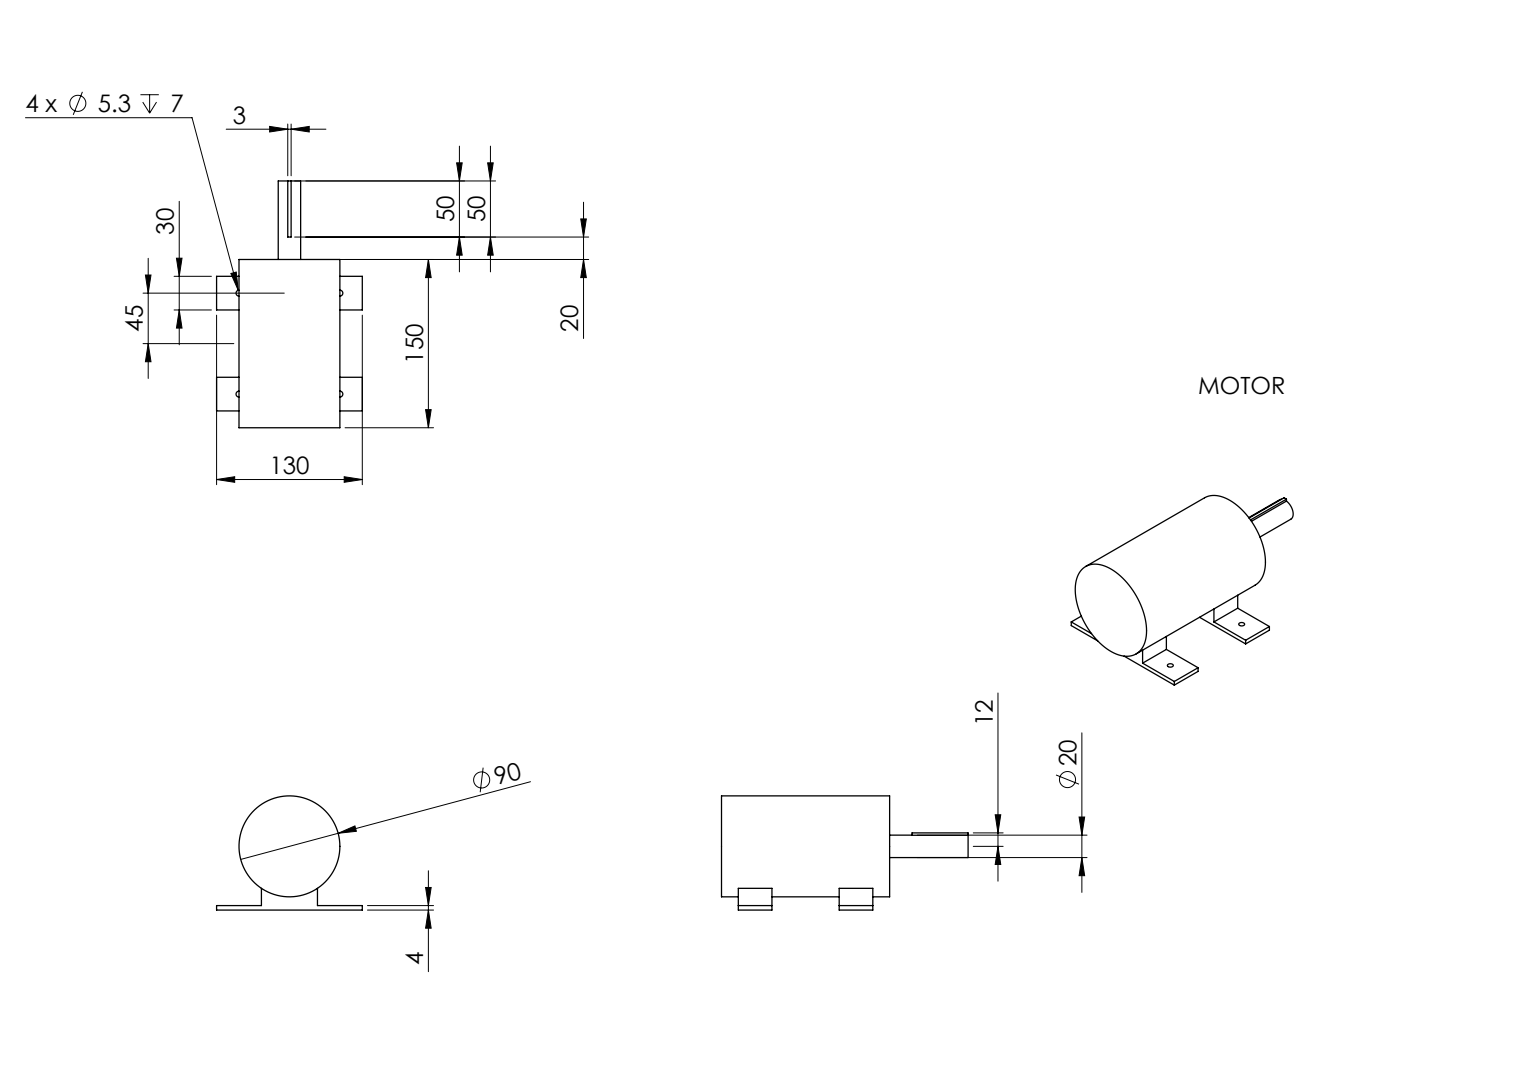
ISO-10303-21;
HEADER;
FILE_DESCRIPTION (('STEP AP214'),
    '1' );
FILE_NAME ('motor.step',
    '2026-10-31T03:46:07',
    ( '' ),
    ( '' ),
    'SwSTEP 2.0',
    'SolidWorks 2026',
    '' );
FILE_SCHEMA (( 'AUTOMOTIVE_DESIGN' ));
ENDSEC;

DATA;
#31=EDGE_CURVE ( 'NONE', #18619, #12627, #9184, .T. ) ;
#51=DIRECTION ( 'NONE',  ( -0.000000000000000000, 3.469446951953613794E-15, 1.000000000000000000 ) ) ;
#52=VERTEX_POINT ( 'NONE', #18122 ) ;
#60=EDGE_CURVE ( 'NONE', #21739, #840, #11018, .T. ) ;
#75=ORIENTED_EDGE ( 'NONE', *, *, #4902, .T. ) ;
#109=AXIS2_PLACEMENT_3D ( 'NONE', #8463, #1435, #15716 ) ;
#182=ADVANCED_FACE ( 'NONE', ( #22679 ), #11370, .F. ) ;
#186=DIRECTION ( 'NONE',  ( 0.000000000000000000, 0.000000000000000000, 1.000000000000000000 ) ) ;
#214=FACE_BOUND ( 'NONE', #6282, .T. ) ;
#228=CARTESIAN_POINT ( 'NONE',  ( -44.99999999999995026, -52.79999999999969873, 50.00000000000018474 ) ) ;
#267=EDGE_CURVE ( 'NONE', #8364, #19016, #14886, .T. ) ;
#271=EDGE_CURVE ( 'NONE', #15472, #22598, #15342, .T. ) ;
#296=VECTOR ( 'NONE', #1760, 1000.000000000000000 ) ;
#300=DIRECTION ( 'NONE',  ( 1.000000000000000000, 3.202566417187951028E-16, 6.405132834375902056E-16 ) ) ;
#324=DIRECTION ( 'NONE',  ( 0.000000000000000000, 0.000000000000000000, 1.000000000000000000 ) ) ;
#328=DIRECTION ( 'NONE',  ( 0.000000000000000000, 0.000000000000000000, 1.000000000000000000 ) ) ;
#332=ORIENTED_EDGE ( 'NONE', *, *, #16929, .T. ) ;
#347=LINE ( 'NONE', #14855, #18432 ) ;
#354=MECHANICAL_DESIGN_GEOMETRIC_PRESENTATION_REPRESENTATION('',(#10787),#11568);
#418=DIRECTION ( 'NONE',  ( 1.000000000000000000, 3.202566417187951028E-16, 6.405132834375902056E-16 ) ) ;
#436=VERTEX_POINT ( 'NONE', #17740 ) ;
#447=DIRECTION ( 'NONE',  ( 0.000000000000000000, 0.000000000000000000, 1.000000000000000000 ) ) ;
#475=CARTESIAN_POINT ( 'NONE',  ( -64.99999999999995737, -56.79999999999964899, 65.00000000000018474 ) ) ;
#486=VECTOR ( 'NONE', #22174, 1000.000000000000000 ) ;
#488=EDGE_CURVE ( 'NONE', #4511, #21370, #19433, .T. ) ;
#514=ORIENTED_EDGE ( 'NONE', *, *, #11865, .F. ) ;
#573=FACE_OUTER_BOUND ( 'NONE', #17478, .T. ) ;
#585=EDGE_CURVE ( 'NONE', #16285, #2501, #3259, .T. ) ;
#591=ORIENTED_EDGE ( 'NONE', *, *, #17311, .T. ) ;
#622=EDGE_LOOP ( 'NONE', ( #22663, #20160, #16621, #5819 ) ) ;
#695=AXIS2_PLACEMENT_3D ( 'NONE', #11043, #18024, #7144 ) ;
#700=ORIENTED_EDGE ( 'NONE', *, *, #8357, .T. ) ;
#712=LINE ( 'NONE', #4213, #4849 ) ;
#713=EDGE_CURVE ( 'NONE', #9956, #13794, #10236, .T. ) ;
#721=VECTOR ( 'NONE', #17814, 1000.000000000000000 ) ;
#731=ORIENTED_EDGE ( 'NONE', *, *, #5331, .T. ) ;
#753=UNCERTAINTY_MEASURE_WITH_UNIT (LENGTH_MEASURE( 1.000000000000000082E-05 ), #23433, 'distance_accuracy_value', 'NONE');
#754=FACE_OUTER_BOUND ( 'NONE', #19293, .T. ) ;
#786=LINE ( 'NONE', #9977, #23718 ) ;
#797=FACE_OUTER_BOUND ( 'NONE', #2972, .T. ) ;
#840=VERTEX_POINT ( 'NONE', #23717 ) ;
#894=DIRECTION ( 'NONE',  ( 0.000000000000000000, -1.000000000000000000, 3.392348130799088816E-15 ) ) ;
#943=ORIENTED_EDGE ( 'NONE', *, *, #1344, .F. ) ;
#989=DIRECTION ( 'NONE',  ( 0.000000000000000000, 0.000000000000000000, 1.000000000000000000 ) ) ;
#993=EDGE_LOOP ( 'NONE', ( #23590, #14200 ) ) ;
#1019=ORIENTED_EDGE ( 'NONE', *, *, #13645, .T. ) ;
#1061=EDGE_LOOP ( 'NONE', ( #11544, #14347, #943, #7992 ) ) ;
#1081=DIRECTION ( 'NONE',  ( 1.000000000000000000, 3.736327486719276364E-16, 1.067522139062650425E-16 ) ) ;
#1090=DIRECTION ( 'NONE',  ( 1.000000000000000000, 3.469446951953598905E-16, -4.625929269271499719E-16 ) ) ;
#1094=VECTOR ( 'NONE', #15458, 1000.000000000000000 ) ;
#1097=CARTESIAN_POINT ( 'NONE',  ( 25.00000000000001421, -37.41657386773940885, 125.0000000000001705 ) ) ;
#1101=DIRECTION ( 'NONE',  ( 3.202566417187928841E-16, -1.000000000000000000, 3.469446951953614583E-15 ) ) ;
#1155=ADVANCED_FACE ( 'NONE', ( #19690 ), #10664, .F. ) ;
#1156=VERTEX_POINT ( 'NONE', #21271 ) ;
#1180=CARTESIAN_POINT ( 'NONE',  ( 65.00000000000001421, -52.79999999999938609, 125.0000000000002274 ) ) ;
#1201=CARTESIAN_POINT ( 'NONE',  ( -44.99999999999995026, -52.79999999999969162, 52.65000000000017621 ) ) ;
#1218=ADVANCED_FACE ( 'NONE', ( #7472 ), #7018, .T. ) ;
#1228=DIRECTION ( 'NONE',  ( -0.000000000000000000, -0.000000000000000000, -1.000000000000000000 ) ) ;
#1234=ORIENTED_EDGE ( 'NONE', *, *, #20465, .F. ) ;
#1239=DIRECTION ( 'NONE',  ( 0.000000000000000000, 2.618450529776326854E-15, 1.000000000000000000 ) ) ;
#1245=DIRECTION ( 'NONE',  ( 3.736327486719275871E-16, -1.000000000000000000, 3.469446951953613794E-15 ) ) ;
#1257=VERTEX_POINT ( 'NONE', #22201 ) ;
#1270=CARTESIAN_POINT ( 'NONE',  ( 1.500000000000000000, 0.000000000000000000, 0.000000000000000000 ) ) ;
#1273=FACE_OUTER_BOUND ( 'NONE', #8704, .T. ) ;
#1277=VERTEX_POINT ( 'NONE', #3856 ) ;
#1292=ORIENTED_EDGE ( 'NONE', *, *, #17778, .T. ) ;
#1324=ORIENTED_EDGE ( 'NONE', *, *, #4746, .T. ) ;
#1344=EDGE_CURVE ( 'NONE', #18619, #4703, #7733, .T. ) ;
#1346=EDGE_CURVE ( 'NONE', #19016, #7096, #712, .T. ) ;
#1353=EDGE_LOOP ( 'NONE', ( #21943, #75 ) ) ;
#1376=ADVANCED_FACE ( 'NONE', ( #19177 ), #11869, .T. ) ;
#1379=ADVANCED_FACE ( 'NONE', ( #11635 ), #2640, .F. ) ;
#1417=PLANE ( 'NONE',  #12387 ) ;
#1424=ORIENTED_EDGE ( 'NONE', *, *, #19677, .F. ) ;
#1425=VECTOR ( 'NONE', #2146, 1000.000000000000000 ) ;
#1426=CARTESIAN_POINT ( 'NONE',  ( 25.00000000000004263, -37.41657386773938754, 65.00000000000018474 ) ) ;
#1435=DIRECTION ( 'NONE',  ( 0.000000000000000000, 0.000000000000000000, 1.000000000000000000 ) ) ;
#1443=EDGE_CURVE ( 'NONE', #4246, #14920, #21250, .T. ) ;
#1489=ORIENTED_EDGE ( 'NONE', *, *, #11624, .T. ) ;
#1499=AXIS2_PLACEMENT_3D ( 'NONE', #3288, #4753, #2922 ) ;
#1592=VERTEX_POINT ( 'NONE', #1660 ) ;
#1593=ORIENTED_EDGE ( 'NONE', *, *, #2778, .F. ) ;
#1610=CARTESIAN_POINT ( 'NONE',  ( -44.99999999999997868, -52.79999999999939320, 137.3500000000001648 ) ) ;
#1639=EDGE_CURVE ( 'NONE', #1592, #2833, #13352, .T. ) ;
#1660=CARTESIAN_POINT ( 'NONE',  ( 45.00000000000002132, -56.79999999999935767, 137.3500000000002217 ) ) ;
#1662=AXIS2_PLACEMENT_3D ( 'NONE', #5057, #9144, #22047 ) ;
#1664=EDGE_CURVE ( 'NONE', #21370, #4532, #16298, .T. ) ;
#1673=CARTESIAN_POINT ( 'NONE',  ( 45.00000000000004974, -52.79999999999967741, 47.35000000000018616 ) ) ;
#1691=LINE ( 'NONE', #1933, #20050 ) ;
#1707=CARTESIAN_POINT ( 'NONE',  ( -44.99999999999997868, -52.79999999999938609, 140.0000000000001421 ) ) ;
#1752=CIRCLE ( 'NONE', #22195, 2.649999999999999467 ) ;
#1759=CARTESIAN_POINT ( 'NONE',  ( -1.500000000000000000, 12.00000000000000000, -50.00000000000000000 ) ) ;
#1760=DIRECTION ( 'NONE',  ( -1.000000000000000000, 0.000000000000000000, 0.000000000000000000 ) ) ;
#1789=PRODUCT_DEFINITION_CONTEXT ( 'detailed design', #19235, 'design' ) ;
#1792=CARTESIAN_POINT ( 'NONE',  ( -44.99999999999995026, -52.79999999999969873, 50.00000000000018474 ) ) ;
#1800=ADVANCED_FACE ( 'NONE', ( #214, #573 ), #4314, .F. ) ;
#1808=CYLINDRICAL_SURFACE ( 'NONE', #23222, 2.649999999999999467 ) ;
#1813=DIRECTION ( 'NONE',  ( 1.751623080406021339E-46, 3.469446951953613794E-15, 1.000000000000000000 ) ) ;
#1828=LINE ( 'NONE', #5350, #21940 ) ;
#1839=CARTESIAN_POINT ( 'NONE',  ( -1.500000000000000000, 9.886859966642592923, -50.00000000000000000 ) ) ;
#1849=CARTESIAN_POINT ( 'NONE',  ( 45.00000000000000711, 5.510910596163090344E-15, 169.9999999999999716 ) ) ;
#1863=AXIS2_PLACEMENT_3D ( 'NONE', #5506, #11334, #20339 ) ;
#1865=LINE ( 'NONE', #21914, #7643 ) ;
#1875=ORIENTED_EDGE ( 'NONE', *, *, #2102, .F. ) ;
#1895=CARTESIAN_POINT ( 'NONE',  ( 45.00000000000004974, -52.79999999999966320, 52.65000000000017621 ) ) ;
#1905=ADVANCED_FACE ( 'NONE', ( #1273 ), #8190, .F. ) ;
#1933=CARTESIAN_POINT ( 'NONE',  ( -24.99999999999995381, -52.79999999999975557, 35.00000000000017764 ) ) ;
#1940=EDGE_CURVE ( 'NONE', #10258, #9956, #8997, .T. ) ;
#1943=LINE ( 'NONE', #5686, #11472 ) ;
#1968=CARTESIAN_POINT ( 'NONE',  ( 45.00000000000002132, -52.79999999999935767, 142.6500000000002046 ) ) ;
#2007=DIRECTION ( 'NONE',  ( 0.000000000000000000, -3.469446951953613794E-15, -1.000000000000000000 ) ) ;
#2016=VECTOR ( 'NONE', #23551, 1000.000000000000000 ) ;
#2045=DIRECTION ( 'NONE',  ( 0.000000000000000000, 2.618450529776313049E-15, 1.000000000000000000 ) ) ;
#2057=AXIS2_PLACEMENT_3D ( 'NONE', #14966, #22065, #4060 ) ;
#2074=ORIENTED_EDGE ( 'NONE', *, *, #31, .T. ) ;
#2102=EDGE_CURVE ( 'NONE', #10287, #52, #11208, .T. ) ;
#2145=CARTESIAN_POINT ( 'NONE',  ( 0.000000000000000000, 0.000000000000000000, 155.0000000000000284 ) ) ;
#2146=DIRECTION ( 'NONE',  ( 1.751623080406021339E-46, 3.469446951953613794E-15, 1.000000000000000000 ) ) ;
#2152=CYLINDRICAL_SURFACE ( 'NONE', #19096, 2.649999999999999467 ) ;
#2168=CARTESIAN_POINT ( 'NONE',  ( 45.00000000000004974, -52.79999999999966320, 52.65000000000018332 ) ) ;
#2206=AXIS2_PLACEMENT_3D ( 'NONE', #13977, #1245, #21179 ) ;
#2244=EDGE_LOOP ( 'NONE', ( #17085, #2250, #21077, #7054 ) ) ;
#2250=ORIENTED_EDGE ( 'NONE', *, *, #14976, .F. ) ;
#2322=PRODUCT_DEFINITION_FORMATION_WITH_SPECIFIED_SOURCE ( 'ANY', '', #3218, .NOT_KNOWN. ) ;
#2366=CARTESIAN_POINT ( 'NONE',  ( 25.00000000000002132, -52.79999999999942162, 125.0000000000001990 ) ) ;
#2398=DIRECTION ( 'NONE',  ( 3.736327486719275871E-16, -1.000000000000000000, 3.469446951953614189E-15 ) ) ;
#2436=DIRECTION ( 'NONE',  ( -0.000000000000000000, 1.000000000000000000, -3.469446951953613794E-15 ) ) ;
#2437=EDGE_LOOP ( 'NONE', ( #12043, #17343, #8968, #13517, #4232, #20219, #1875, #17937 ) ) ;
#2464=CIRCLE ( 'NONE', #9037, 2.649999999999985700 ) ;
#2465=DIRECTION ( 'NONE',  ( -1.000000000000000000, -3.202566417187951028E-16, -6.405132834375902056E-16 ) ) ;
#2501=VERTEX_POINT ( 'NONE', #20080 ) ;
#2505=FACE_OUTER_BOUND ( 'NONE', #10784, .T. ) ;
#2522=DIRECTION ( 'NONE',  ( 0.000000000000000000, 0.000000000000000000, 1.000000000000000000 ) ) ;
#2528=EDGE_LOOP ( 'NONE', ( #23738, #21267 ) ) ;
#2614=DIRECTION ( 'NONE',  ( -4.625929269271485914E-16, -3.469446951953614583E-15, -1.000000000000000000 ) ) ;
#2633=ORIENTED_EDGE ( 'NONE', *, *, #5098, .T. ) ;
#2637=CARTESIAN_POINT ( 'NONE',  ( -24.99999999999998579, -37.41657386773942306, 169.9999999999999716 ) ) ;
#2640=PLANE ( 'NONE',  #17162 ) ;
#2658=EDGE_CURVE ( 'NONE', #2501, #12643, #22364, .T. ) ;
#2679=ORIENTED_EDGE ( 'NONE', *, *, #6053, .T. ) ;
#2694=AXIS2_PLACEMENT_3D ( 'NONE', #9686, #4584, #15123 ) ;
#2762=DIRECTION ( 'NONE',  ( -0.000000000000000000, 1.000000000000000000, -3.469446951953613794E-15 ) ) ;
#2766=DIRECTION ( 'NONE',  ( -0.000000000000000000, 1.000000000000000000, -3.469446951953613794E-15 ) ) ;
#2778=EDGE_CURVE ( 'NONE', #4532, #8574, #10433, .T. ) ;
#2833=VERTEX_POINT ( 'NONE', #14730 ) ;
#2836=DIRECTION ( 'NONE',  ( 0.000000000000000000, -2.618450529776313049E-15, -1.000000000000000000 ) ) ;
#2885=ORIENTED_EDGE ( 'NONE', *, *, #22707, .F. ) ;
#2898=DIRECTION ( 'NONE',  ( 0.000000000000000000, -2.618450529776326854E-15, -1.000000000000000000 ) ) ;
#2899=CARTESIAN_POINT ( 'NONE',  ( 25.00000000000004974, -52.79999999999973426, 35.00000000000017764 ) ) ;
#2918=CARTESIAN_POINT ( 'NONE',  ( -1.500000000000000000, 12.00000000000000000, 0.000000000000000000 ) ) ;
#2920=EDGE_CURVE ( 'NONE', #1277, #23309, #20491, .T. ) ;
#2922=DIRECTION ( 'NONE',  ( -1.000000000000000000, 0.000000000000000000, 0.000000000000000000 ) ) ;
#2941=ORIENTED_EDGE ( 'NONE', *, *, #10411, .F. ) ;
#2972=EDGE_LOOP ( 'NONE', ( #19259, #16489, #3704, #1292 ) ) ;
#2979=DIRECTION ( 'NONE',  ( 2.238759164535664589E-46, 3.469446951953614189E-15, 1.000000000000000000 ) ) ;
#2982=VERTEX_POINT ( 'NONE', #18663 ) ;
#2991=CARTESIAN_POINT ( 'NONE',  ( 1.500000000000000000, 12.00000000000000000, 0.000000000000000000 ) ) ;
#3005=AXIS2_PLACEMENT_3D ( 'NONE', #7570, #5878, #2007 ) ;
#3007=CIRCLE ( 'NONE', #23458, 2.649999999999999467 ) ;
#3045=DIRECTION ( 'NONE',  ( 0.000000000000000000, 0.000000000000000000, 1.000000000000000000 ) ) ;
#3113=VERTEX_POINT ( 'NONE', #8546 ) ;
#3124=SHAPE_REPRESENTATION ( 'motor', ( #11210 ), #7665 ) ;
#3189=DIRECTION ( 'NONE',  ( 3.736327486719275871E-16, -1.000000000000000000, 3.469446951953613794E-15 ) ) ;
#3218=PRODUCT ( 'motor', 'motor', '', ( #7579 ) ) ;
#3234=ORIENTED_EDGE ( 'NONE', *, *, #21969, .F. ) ;
#3247=CARTESIAN_POINT ( 'NONE',  ( -24.99999999999998934, 45.00100000000031031, 34.99999999999983658 ) ) ;
#3254=DIRECTION ( 'NONE',  ( -0.000000000000000000, 1.000000000000000000, -3.469446951953613794E-15 ) ) ;
#3259=CIRCLE ( 'NONE', #12952, 45.00000000000000711 ) ;
#3272=CIRCLE ( 'NONE', #16782, 45.00000000000000711 ) ;
#3281=CYLINDRICAL_SURFACE ( 'NONE', #20382, 45.00000000000000711 ) ;
#3288=CARTESIAN_POINT ( 'NONE',  ( 0.000000000000000000, 0.000000000000000000, 169.9999999999999716 ) ) ;
#3294=DIRECTION ( 'NONE',  ( 1.000000000000000000, 0.000000000000000000, 0.000000000000000000 ) ) ;
#3296=LINE ( 'NONE', #1610, #20557 ) ;
#3309=EDGE_LOOP ( 'NONE', ( #10169, #7031, #1019, #15364 ) ) ;
#3310=ADVANCED_FACE ( 'NONE', ( #23331 ), #14321, .F. ) ;
#3324=ORIENTED_EDGE ( 'NONE', *, *, #3934, .T. ) ;
#3334=ADVANCED_FACE ( 'NONE', ( #23094 ), #12517, .T. ) ;
#3365=ADVANCED_FACE ( 'NONE', ( #4743 ), #3281, .T. ) ;
#3374=ADVANCED_FACE ( 'NONE', ( #12272 ), #10198, .F. ) ;
#3382=AXIS2_PLACEMENT_3D ( 'NONE', #13638, #9741, #894 ) ;
#3415=VERTEX_POINT ( 'NONE', #23246 ) ;
#3427=VECTOR ( 'NONE', #7829, 1000.000000000000000 ) ;
#3495=SURFACE_STYLE_USAGE ( .BOTH. , #5756 ) ;
#3528=ORIENTED_EDGE ( 'NONE', *, *, #4495, .F. ) ;
#3529=DIRECTION ( 'NONE',  ( 3.736327486719275871E-16, -1.000000000000000000, 3.469446951953613794E-15 ) ) ;
#3538=EDGE_CURVE ( 'NONE', #12643, #17916, #11599, .T. ) ;
#3565=EDGE_LOOP ( 'NONE', ( #5410, #19936, #9737, #16180 ) ) ;
#3574=EDGE_CURVE ( 'NONE', #8832, #13580, #22258, .T. ) ;
#3575=ORIENTED_EDGE ( 'NONE', *, *, #7698, .T. ) ;
#3578=EDGE_LOOP ( 'NONE', ( #16303, #3575, #14895, #19374 ) ) ;
#3589=DIRECTION ( 'NONE',  ( -0.000000000000000000, 1.000000000000000000, -3.469446951953613794E-15 ) ) ;
#3592=CARTESIAN_POINT ( 'NONE',  ( 65.00000000000004263, -52.79999999999959925, 65.00000000000018474 ) ) ;
#3594=VECTOR ( 'NONE', #20916, 1000.000000000000000 ) ;
#3673=AXIS2_PLACEMENT_3D ( 'NONE', #18231, #10908, #20269 ) ;
#3681=ORIENTED_EDGE ( 'NONE', *, *, #22989, .F. ) ;
#3695=CARTESIAN_POINT ( 'NONE',  ( 45.00000000000002132, -56.79999999999935056, 140.0000000000001990 ) ) ;
#3704=ORIENTED_EDGE ( 'NONE', *, *, #713, .T. ) ;
#3719=CARTESIAN_POINT ( 'NONE',  ( 65.00000000000005684, -52.79999999999970584, 35.00000000000017764 ) ) ;
#3724=EDGE_LOOP ( 'NONE', ( #11287, #11752 ) ) ;
#3744=ORIENTED_EDGE ( 'NONE', *, *, #7934, .F. ) ;
#3768=CARTESIAN_POINT ( 'NONE',  ( 45.00000000000002132, -52.79999999999936477, 137.3500000000002217 ) ) ;
#3769=DIRECTION ( 'NONE',  ( 1.000000000000000000, 0.000000000000000000, 0.000000000000000000 ) ) ;
#3773=CARTESIAN_POINT ( 'NONE',  ( -44.99999999999997868, -56.79999999999937188, 142.6500000000001478 ) ) ;
#3786=ORIENTED_EDGE ( 'NONE', *, *, #6661, .T. ) ;
#3789=DIRECTION ( 'NONE',  ( 0.000000000000000000, 0.000000000000000000, 1.000000000000000000 ) ) ;
#3840=VECTOR ( 'NONE', #7258, 1000.000000000000000 ) ;
#3847=ADVANCED_FACE ( 'NONE', ( #12418, #10696, #21659 ), #5115, .T. ) ;
#3853=CARTESIAN_POINT ( 'NONE',  ( 25.00000000000002132, -52.79999999999942162, 125.0000000000001990 ) ) ;
#3856=CARTESIAN_POINT ( 'NONE',  ( 65.00000000000002842, -52.79999999999929372, 155.0000000000002274 ) ) ;
#3881=EDGE_LOOP ( 'NONE', ( #19327, #2633, #15079, #19810 ) ) ;
#3924=SHAPE_REPRESENTATION_RELATIONSHIP ( 'NONE' , 'NONE' ,  #3124, #22256 ) ;
#3928=EDGE_CURVE ( 'NONE', #12485, #6553, #1828, .T. ) ;
#3934=EDGE_CURVE ( 'NONE', #12627, #22432, #11178, .T. ) ;
#3962=FACE_OUTER_BOUND ( 'NONE', #3881, .T. ) ;
#3963=EDGE_CURVE ( 'NONE', #8364, #436, #7509, .T. ) ;
#3986=VECTOR ( 'NONE', #10399, 1000.000000000000000 ) ;
#4058=AXIS2_PLACEMENT_3D ( 'NONE', #14297, #1090, #15857 ) ;
#4060=DIRECTION ( 'NONE',  ( 0.000000000000000000, 2.618450529776326854E-15, 1.000000000000000000 ) ) ;
#4078=DIRECTION ( 'NONE',  ( -2.238759164535664589E-46, -3.469446951953614189E-15, -1.000000000000000000 ) ) ;
#4142=VERTEX_POINT ( 'NONE', #23428 ) ;
#4193=ORIENTED_EDGE ( 'NONE', *, *, #9622, .T. ) ;
#4213=CARTESIAN_POINT ( 'NONE',  ( -25.00000000000001776, 45.00100000000072953, 154.9999999999998579 ) ) ;
#4226=AXIS2_PLACEMENT_3D ( 'NONE', #20020, #12709, #7213 ) ;
#4227=CARTESIAN_POINT ( 'NONE',  ( -64.99999999999998579, -52.79999999999942872, 125.0000000000001421 ) ) ;
#4232=ORIENTED_EDGE ( 'NONE', *, *, #11663, .T. ) ;
#4244=CIRCLE ( 'NONE', #5411, 2.649999999999985700 ) ;
#4246=VERTEX_POINT ( 'NONE', #1097 ) ;
#4254=ADVANCED_FACE ( 'NONE', ( #23197 ), #12254, .T. ) ;
#4307=LINE ( 'NONE', #16859, #6183 ) ;
#4312=DIRECTION ( 'NONE',  ( 1.000000000000000000, 0.000000000000000000, 0.000000000000000000 ) ) ;
#4314=PLANE ( 'NONE',  #3005 ) ;
#4382=ORIENTED_EDGE ( 'NONE', *, *, #488, .T. ) ;
#4398=EDGE_LOOP ( 'NONE', ( #9314, #14380, #9069, #16829 ) ) ;
#4423=CARTESIAN_POINT ( 'NONE',  ( 25.00000000000001066, 45.00100000000033162, 34.99999999999983658 ) ) ;
#4442=AXIS2_PLACEMENT_3D ( 'NONE', #18688, #9678, #7963 ) ;
#4458=CARTESIAN_POINT ( 'NONE',  ( -65.00000000000000000, -56.79999999999932925, 155.0000000000001705 ) ) ;
#4459=ORIENTED_EDGE ( 'NONE', *, *, #3574, .T. ) ;
#4467=ADVANCED_FACE ( 'NONE', ( #3962 ), #2152, .F. ) ;
#4479=AXIS2_PLACEMENT_3D ( 'NONE', #20915, #2436, #9708 ) ;
#4495=EDGE_CURVE ( 'NONE', #1277, #5510, #21124, .T. ) ;
#4511=VERTEX_POINT ( 'NONE', #15480 ) ;
#4531=CARTESIAN_POINT ( 'NONE',  ( 1.500000000000000000, 12.00000000000000000, 0.000000000000000000 ) ) ;
#4532=VERTEX_POINT ( 'NONE', #1201 ) ;
#4541=DIRECTION ( 'NONE',  ( 1.000000000000000000, 0.000000000000000000, 0.000000000000000000 ) ) ;
#4552=EDGE_CURVE ( 'NONE', #12588, #21739, #12230, .T. ) ;
#4584=DIRECTION ( 'NONE',  ( 3.736327486719275871E-16, -1.000000000000000000, 3.469446951953613794E-15 ) ) ;
#4605=LINE ( 'NONE', #6411, #8756 ) ;
#4619=CARTESIAN_POINT ( 'NONE',  ( -24.99999999999996092, -37.41657386773943728, 35.00000000000013500 ) ) ;
#4640=DIRECTION ( 'NONE',  ( -0.000000000000000000, -0.000000000000000000, -1.000000000000000000 ) ) ;
#4650=AXIS2_PLACEMENT_3D ( 'NONE', #228, #13301, #6137 ) ;
#4683=LINE ( 'NONE', #13900, #23065 ) ;
#4703=VERTEX_POINT ( 'NONE', #1426 ) ;
#4713=CARTESIAN_POINT ( 'NONE',  ( -64.99999999999995737, -52.79999999999965610, 65.00000000000017053 ) ) ;
#4714=( LENGTH_UNIT ( ) NAMED_UNIT ( * ) SI_UNIT ( .MILLI., .METRE. ) );
#4743=FACE_OUTER_BOUND ( 'NONE', #20923, .T. ) ;
#4744=DIRECTION ( 'NONE',  ( -1.000000000000000000, 0.000000000000000000, 0.000000000000000000 ) ) ;
#4746=EDGE_CURVE ( 'NONE', #2501, #16285, #3272, .T. ) ;
#4753=DIRECTION ( 'NONE',  ( -0.000000000000000000, -0.000000000000000000, -1.000000000000000000 ) ) ;
#4761=EDGE_CURVE ( 'NONE', #15959, #10287, #786, .T. ) ;
#4788=CARTESIAN_POINT ( 'NONE',  ( 45.00000000000004974, -56.79999999999966320, 52.65000000000019753 ) ) ;
#4797=DIRECTION ( 'NONE',  ( -1.000000000000000000, -3.469446951953630952E-16, -4.625929269271472109E-16 ) ) ;
#4804=ORIENTED_EDGE ( 'NONE', *, *, #19808, .T. ) ;
#4818=DIRECTION ( 'NONE',  ( 0.000000000000000000, 2.618450529776313049E-15, 1.000000000000000000 ) ) ;
#4832=FACE_OUTER_BOUND ( 'NONE', #20243, .T. ) ;
#4849=VECTOR ( 'NONE', #8099, 1000.000000000000000 ) ;
#4850=CARTESIAN_POINT ( 'NONE',  ( -64.99999999999997158, -52.79999999999974847, 35.00000000000017764 ) ) ;
#4869=CARTESIAN_POINT ( 'NONE',  ( 1.500000000000000000, 0.000000000000000000, 0.000000000000000000 ) ) ;
#4873=LINE ( 'NONE', #2918, #21876 ) ;
#4874=ORIENTED_EDGE ( 'NONE', *, *, #10945, .T. ) ;
#4880=CARTESIAN_POINT ( 'NONE',  ( -24.99999999999998579, -37.41657386773942306, 155.0000000000001705 ) ) ;
#4902=EDGE_CURVE ( 'NONE', #13580, #4142, #13759, .T. ) ;
#4903=VECTOR ( 'NONE', #2398, 1000.000000000000000 ) ;
#4956=AXIS2_PLACEMENT_3D ( 'NONE', #15563, #22889, #6357 ) ;
#4972=AXIS2_PLACEMENT_3D ( 'NONE', #19995, #6732, #9025 ) ;
#5013=ORIENTED_EDGE ( 'NONE', *, *, #13507, .F. ) ;
#5017=VECTOR ( 'NONE', #17639, 1000.000000000000000 ) ;
#5057=CARTESIAN_POINT ( 'NONE',  ( 0.000000000000000000, 0.000000000000000000, 0.000000000000000000 ) ) ;
#5058=VERTEX_POINT ( 'NONE', #21773 ) ;
#5098=EDGE_CURVE ( 'NONE', #23584, #18606, #1752, .T. ) ;
#5109=DIRECTION ( 'NONE',  ( 1.000000000000000000, 0.000000000000000000, 0.000000000000000000 ) ) ;
#5115=CYLINDRICAL_SURFACE ( 'NONE', #1499, 45.00000000000000711 ) ;
#5118=CIRCLE ( 'NONE', #12495, 2.649999999999985700 ) ;
#5180=DIRECTION ( 'NONE',  ( 3.469446951953614682E-16, -1.000000000000000000, 3.483493295888648978E-15 ) ) ;
#5192=EDGE_CURVE ( 'NONE', #13453, #2982, #16348, .T. ) ;
#5195=ORIENTED_EDGE ( 'NONE', *, *, #31, .F. ) ;
#5196=ADVANCED_FACE ( 'NONE', ( #754 ), #13714, .F. ) ;
#5205=VECTOR ( 'NONE', #8406, 1000.000000000000000 ) ;
#5232=ADVANCED_FACE ( 'NONE', ( #18970 ), #7881, .F. ) ;
#5241=ORIENTED_EDGE ( 'NONE', *, *, #2778, .T. ) ;
#5322=EDGE_CURVE ( 'NONE', #9373, #8692, #4244, .T. ) ;
#5331=EDGE_CURVE ( 'NONE', #21739, #12627, #10554, .T. ) ;
#5350=CARTESIAN_POINT ( 'NONE',  ( -24.99999999999998934, 45.00100000000031031, 34.99999999999983658 ) ) ;
#5410=ORIENTED_EDGE ( 'NONE', *, *, #23493, .T. ) ;
#5411=AXIS2_PLACEMENT_3D ( 'NONE', #8487, #1101, #2898 ) ;
#5414=CARTESIAN_POINT ( 'NONE',  ( 1.500000000000000000, 12.00000000000000000, -50.00000000000000000 ) ) ;
#5434=CARTESIAN_POINT ( 'NONE',  ( 45.00000000000002132, -56.79999999999935056, 140.0000000000001990 ) ) ;
#5463=ORIENTED_EDGE ( 'NONE', *, *, #14844, .T. ) ;
#5506=CARTESIAN_POINT ( 'NONE',  ( 0.000000000000000000, 0.000000000000000000, -50.00000000000000000 ) ) ;
#5510=VERTEX_POINT ( 'NONE', #13088 ) ;
#5514=EDGE_CURVE ( 'NONE', #13453, #19560, #18478, .T. ) ;
#5579=EDGE_CURVE ( 'NONE', #6553, #21767, #1691, .T. ) ;
#5681=FACE_OUTER_BOUND ( 'NONE', #14860, .T. ) ;
#5684=CARTESIAN_POINT ( 'NONE',  ( -24.99999999999995381, -52.79999999999965610, 65.00000000000018474 ) ) ;
#5686=CARTESIAN_POINT ( 'NONE',  ( -24.99999999999998224, -52.79999999999944293, 125.0000000000001990 ) ) ;
#5695=EDGE_LOOP ( 'NONE', ( #20282, #23163 ) ) ;
#5708=CARTESIAN_POINT ( 'NONE',  ( -64.99999999999997158, -56.79999999999975557, 35.00000000000019185 ) ) ;
#5753=AXIS2_PLACEMENT_3D ( 'NONE', #17540, #989, #12411 ) ;
#5756=SURFACE_SIDE_STYLE ('',( #15605 ) ) ;
#5764=CIRCLE ( 'NONE', #19246, 45.00000000000000711 ) ;
#5793=VECTOR ( 'NONE', #23523, 1000.000000000000000 ) ;
#5819=ORIENTED_EDGE ( 'NONE', *, *, #7398, .T. ) ;
#5870=DIRECTION ( 'NONE',  ( 1.000000000000000000, 3.736327486719276364E-16, 1.067522139062650425E-16 ) ) ;
#5878=DIRECTION ( 'NONE',  ( 3.736327486719275871E-16, -1.000000000000000000, 3.469446951953613794E-15 ) ) ;
#5881=ORIENTED_EDGE ( 'NONE', *, *, #17201, .F. ) ;
#5884=CARTESIAN_POINT ( 'NONE',  ( 65.00000000000001421, -52.79999999999938609, 125.0000000000002274 ) ) ;
#5902=DIRECTION ( 'NONE',  ( -0.000000000000000000, 1.000000000000000000, -3.469446951953613794E-15 ) ) ;
#5911=PLANE ( 'NONE',  #2694 ) ;
#5937=AXIS2_PLACEMENT_3D ( 'NONE', #16851, #5982, #9380 ) ;
#5975=DIRECTION ( 'NONE',  ( 1.000000000000000000, 0.000000000000000000, 0.000000000000000000 ) ) ;
#5982=DIRECTION ( 'NONE',  ( 3.202566417187928841E-16, -1.000000000000000000, 3.469446951953614583E-15 ) ) ;
#5995=PLANE ( 'NONE',  #15078 ) ;
#6010=AXIS2_PLACEMENT_3D ( 'NONE', #15147, #20796, #13353 ) ;
#6026=DIRECTION ( 'NONE',  ( 1.000000000000000000, 3.469446951953630952E-16, 4.625929269271474081E-16 ) ) ;
#6028=EDGE_LOOP ( 'NONE', ( #514, #6048 ) ) ;
#6048=ORIENTED_EDGE ( 'NONE', *, *, #23000, .F. ) ;
#6053=EDGE_CURVE ( 'NONE', #8574, #4532, #13948, .T. ) ;
#6094=ADVANCED_FACE ( 'NONE', ( #18795 ), #6372, .F. ) ;
#6099=ORIENTED_EDGE ( 'NONE', *, *, #2102, .T. ) ;
#6137=DIRECTION ( 'NONE',  ( 0.000000000000000000, 2.618450529776319755E-15, 1.000000000000000000 ) ) ;
#6139=DIRECTION ( 'NONE',  ( 0.000000000000000000, 2.618450529776313049E-15, 1.000000000000000000 ) ) ;
#6150=DIRECTION ( 'NONE',  ( 0.000000000000000000, 2.618450529776326854E-15, 1.000000000000000000 ) ) ;
#6183=VECTOR ( 'NONE', #5870, 1000.000000000000000 ) ;
#6199=CARTESIAN_POINT ( 'NONE',  ( -44.99999999999997868, -52.79999999999938609, 140.0000000000001421 ) ) ;
#6271=ORIENTED_EDGE ( 'NONE', *, *, #19425, .T. ) ;
#6276=CARTESIAN_POINT ( 'NONE',  ( 25.00000000000004263, -37.41657386773938754, 169.9999999999999716 ) ) ;
#6282=EDGE_LOOP ( 'NONE', ( #17146, #18799 ) ) ;
#6298=ORIENTED_EDGE ( 'NONE', *, *, #7394, .T. ) ;
#6307=DIRECTION ( 'NONE',  ( 0.000000000000000000, 2.618450529776326854E-15, 1.000000000000000000 ) ) ;
#6357=DIRECTION ( 'NONE',  ( 0.000000000000000000, 0.000000000000000000, -1.000000000000000000 ) ) ;
#6371=AXIS2_PLACEMENT_3D ( 'NONE', #3695, #20015, #11109 ) ;
#6372=PLANE ( 'NONE',  #20441 ) ;
#6396=CARTESIAN_POINT ( 'NONE',  ( -64.99999999999995737, -52.79999999999965610, 65.00000000000017053 ) ) ;
#6411=CARTESIAN_POINT ( 'NONE',  ( -64.99999999999997158, -52.79999999999974847, 35.00000000000017764 ) ) ;
#6483=DIRECTION ( 'NONE',  ( -0.000000000000000000, 1.000000000000000000, -3.469446951953613794E-15 ) ) ;
#6486=FACE_OUTER_BOUND ( 'NONE', #622, .T. ) ;
#6499=ORIENTED_EDGE ( 'NONE', *, *, #1639, .T. ) ;
#6524=ORIENTED_EDGE ( 'NONE', *, *, #13507, .T. ) ;
#6526=DIRECTION ( 'NONE',  ( 0.000000000000000000, 1.000000000000000000, -3.469446951953614189E-15 ) ) ;
#6548=ORIENTED_EDGE ( 'NONE', *, *, #21176, .F. ) ;
#6550=( NAMED_UNIT ( * ) PLANE_ANGLE_UNIT ( ) SI_UNIT ( $, .RADIAN. ) );
#6552=DIRECTION ( 'NONE',  ( -0.000000000000000000, 1.000000000000000000, -3.469446951953613794E-15 ) ) ;
#6553=VERTEX_POINT ( 'NONE', #22273 ) ;
#6564=CARTESIAN_POINT ( 'NONE',  ( 45.00000000000002132, -52.79999999999936477, 137.3500000000002217 ) ) ;
#6612=ADVANCED_FACE ( 'NONE', ( #19130, #6669 ), #12262, .F. ) ;
#6647=DIRECTION ( 'NONE',  ( 0.000000000000000000, 0.000000000000000000, 1.000000000000000000 ) ) ;
#6650=DIRECTION ( 'NONE',  ( -2.238759164535664589E-46, -3.469446951953614189E-15, -1.000000000000000000 ) ) ;
#6661=EDGE_CURVE ( 'NONE', #16285, #17916, #11817, .T. ) ;
#6669=FACE_OUTER_BOUND ( 'NONE', #3565, .T. ) ;
#6673=DIRECTION ( 'NONE',  ( 0.000000000000000000, 0.000000000000000000, 1.000000000000000000 ) ) ;
#6685=DIRECTION ( 'NONE',  ( 0.000000000000000000, 0.000000000000000000, -1.000000000000000000 ) ) ;
#6691=DIRECTION ( 'NONE',  ( 1.000000000000000000, 3.202566417187951028E-16, 6.405132834375902056E-16 ) ) ;
#6732=DIRECTION ( 'NONE',  ( 1.000000000000000000, 3.736327486719275871E-16, -1.296299001029869881E-30 ) ) ;
#6738=CARTESIAN_POINT ( 'NONE',  ( -10.00000000000000000, 1.224646799147353256E-15, -50.00000000000000000 ) ) ;
#6762=ADVANCED_FACE ( 'NONE', ( #5681 ), #1808, .F. ) ;
#6855=FACE_OUTER_BOUND ( 'NONE', #20374, .T. ) ;
#6880=( NAMED_UNIT ( * ) PLANE_ANGLE_UNIT ( ) SI_UNIT ( $, .RADIAN. ) );
#6896=ADVANCED_FACE ( 'NONE', ( #20598, #13053, #10887 ), #9291, .T. ) ;
#6959=AXIS2_PLACEMENT_3D ( 'NONE', #7930, #328, #4541 ) ;
#6964=ORIENTED_EDGE ( 'NONE', *, *, #8123, .F. ) ;
#6973=CARTESIAN_POINT ( 'NONE',  ( 65.00000000000001421, -56.79999999999939320, 125.0000000000002558 ) ) ;
#6978=EDGE_CURVE ( 'NONE', #1156, #17333, #16869, .T. ) ;
#7011=( NAMED_UNIT ( * ) PLANE_ANGLE_UNIT ( ) SI_UNIT ( $, .RADIAN. ) );
#7017=ORIENTED_EDGE ( 'NONE', *, *, #6053, .F. ) ;
#7018=PLANE ( 'NONE',  #3673 ) ;
#7026=DIRECTION ( 'NONE',  ( 3.736327486719275871E-16, -1.000000000000000000, 3.469446951953613794E-15 ) ) ;
#7027=VERTEX_POINT ( 'NONE', #15564 ) ;
#7031=ORIENTED_EDGE ( 'NONE', *, *, #12434, .T. ) ;
#7043=ORIENTED_EDGE ( 'NONE', *, *, #11624, .F. ) ;
#7054=ORIENTED_EDGE ( 'NONE', *, *, #12443, .F. ) ;
#7080=CARTESIAN_POINT ( 'NONE',  ( -44.99999999999997868, -52.79999999999938609, 140.0000000000001421 ) ) ;
#7096=VERTEX_POINT ( 'NONE', #17239 ) ;
#7101=DIRECTION ( 'NONE',  ( -0.000000000000000000, 1.000000000000000000, -3.469446951953613794E-15 ) ) ;
#7131=EDGE_LOOP ( 'NONE', ( #8931, #4459, #7234, #21617, #12795, #17739, #16675, #15139 ) ) ;
#7144=DIRECTION ( 'NONE',  ( 1.000000000000000000, 0.000000000000000000, 0.000000000000000000 ) ) ;
#7172=ADVANCED_FACE ( 'NONE', ( #10414 ), #17870, .T. ) ;
#7213=DIRECTION ( 'NONE',  ( 0.000000000000000000, 2.618450529776319755E-15, 1.000000000000000000 ) ) ;
#7227=ADVANCED_FACE ( 'NONE', ( #10653, #17991 ), #14159, .F. ) ;
#7230=EDGE_CURVE ( 'NONE', #10258, #8832, #20149, .T. ) ;
#7234=ORIENTED_EDGE ( 'NONE', *, *, #10226, .F. ) ;
#7258=DIRECTION ( 'NONE',  ( -4.625929269271485914E-16, 3.469446951953614583E-15, 1.000000000000000000 ) ) ;
#7286=VECTOR ( 'NONE', #19741, 1000.000000000000000 ) ;
#7309=AXIS2_PLACEMENT_3D ( 'NONE', #4869, #4744, #3045 ) ;
#7310=ORIENTED_EDGE ( 'NONE', *, *, #5331, .F. ) ;
#7362=CARTESIAN_POINT ( 'NONE',  ( -44.99999999999995026, -52.79999999999970584, 47.35000000000019327 ) ) ;
#7379=DIRECTION ( 'NONE',  ( 3.736327486719275871E-16, -1.000000000000000000, 3.469446951953614189E-15 ) ) ;
#7394=EDGE_CURVE ( 'NONE', #2833, #1592, #5118, .T. ) ;
#7397=ORIENTED_EDGE ( 'NONE', *, *, #271, .T. ) ;
#7398=EDGE_CURVE ( 'NONE', #12588, #3415, #14612, .T. ) ;
#7400=DIRECTION ( 'NONE',  ( 3.736327486719275871E-16, -1.000000000000000000, 3.469446951953614189E-15 ) ) ;
#7406=EDGE_CURVE ( 'NONE', #23584, #7027, #14739, .T. ) ;
#7430=ADVANCED_FACE ( 'NONE', ( #2505 ), #13564, .F. ) ;
#7459=SHAPE_DEFINITION_REPRESENTATION ( #9034, #3124 ) ;
#7472=FACE_OUTER_BOUND ( 'NONE', #17508, .T. ) ;
#7496=ORIENTED_EDGE ( 'NONE', *, *, #12731, .T. ) ;
#7509=LINE ( 'NONE', #20431, #22316 ) ;
#7510=ORIENTED_EDGE ( 'NONE', *, *, #17353, .F. ) ;
#7537=DIRECTION ( 'NONE',  ( 1.000000000000000000, 0.000000000000000000, 0.000000000000000000 ) ) ;
#7570=CARTESIAN_POINT ( 'NONE',  ( 1.983456134378398743E-14, -52.79999999999986215, 1.831306136874101694E-13 ) ) ;
#7571=CARTESIAN_POINT ( 'NONE',  ( 1.819057724962738742E-14, -56.79999999999984794, 1.970645868709647811E-13 ) ) ;
#7579=PRODUCT_CONTEXT ( 'NONE', #16775, 'mechanical' ) ;
#7643=VECTOR ( 'NONE', #12564, 1000.000000000000000 ) ;
#7648=CIRCLE ( 'NONE', #14618, 45.00000000000000711 ) ;
#7658=EDGE_LOOP ( 'NONE', ( #21127, #22080, #14017, #17202 ) ) ;
#7665=( GEOMETRIC_REPRESENTATION_CONTEXT ( 3 ) GLOBAL_UNCERTAINTY_ASSIGNED_CONTEXT ( ( #22193 ) ) GLOBAL_UNIT_ASSIGNED_CONTEXT ( ( #4714, #6880, #19797 ) ) REPRESENTATION_CONTEXT ( 'NONE', 'WORKASPACE' ) );
#7677=DIRECTION ( 'NONE',  ( -1.000000000000000000, 0.000000000000000000, 0.000000000000000000 ) ) ;
#7695=AXIS2_PLACEMENT_3D ( 'NONE', #18397, #186, #7537 ) ;
#7698=EDGE_CURVE ( 'NONE', #9956, #11870, #15957, .T. ) ;
#7733=LINE ( 'NONE', #6276, #15284 ) ;
#7740=ORIENTED_EDGE ( 'NONE', *, *, #7398, .F. ) ;
#7764=DIRECTION ( 'NONE',  ( -0.000000000000000000, -0.000000000000000000, -1.000000000000000000 ) ) ;
#7829=DIRECTION ( 'NONE',  ( 4.625929269271486900E-16, 3.469446951953614978E-15, 1.000000000000000000 ) ) ;
#7853=STYLED_ITEM('',(#23934),#12608);
#7870=VECTOR ( 'NONE', #12210, 1000.000000000000000 ) ;
#7881=CYLINDRICAL_SURFACE ( 'NONE', #4479, 2.649999999999985700 ) ;
#7924=LINE ( 'NONE', #9634, #11600 ) ;
#7927=VECTOR ( 'NONE', #13927, 1000.000000000000000 ) ;
#7930=CARTESIAN_POINT ( 'NONE',  ( 0.000000000000000000, 0.000000000000000000, 20.00000000000000000 ) ) ;
#7934=EDGE_CURVE ( 'NONE', #3113, #13794, #23358, .T. ) ;
#7947=ORIENTED_EDGE ( 'NONE', *, *, #12443, .T. ) ;
#7953=CARTESIAN_POINT ( 'NONE',  ( 45.00000000000004974, -52.79999999999967031, 50.00000000000018474 ) ) ;
#7963=DIRECTION ( 'NONE',  ( 1.000000000000000000, 0.000000000000000000, -0.000000000000000000 ) ) ;
#7981=ORIENTED_EDGE ( 'NONE', *, *, #12731, .F. ) ;
#7992=ORIENTED_EDGE ( 'NONE', *, *, #13629, .F. ) ;
#8088=AXIS2_PLACEMENT_3D ( 'NONE', #16090, #10676, #8726 ) ;
#8099=DIRECTION ( 'NONE',  ( 3.736327486719275871E-16, -1.000000000000000000, 3.469446951953614189E-15 ) ) ;
#8100=ORIENTED_EDGE ( 'NONE', *, *, #16929, .F. ) ;
#8103=CARTESIAN_POINT ( 'NONE',  ( 45.00000000000004974, -52.79999999999967031, 50.00000000000018474 ) ) ;
#8109=FACE_OUTER_BOUND ( 'NONE', #17856, .T. ) ;
#8123=EDGE_CURVE ( 'NONE', #18606, #21871, #22096, .T. ) ;
#8189=EDGE_CURVE ( 'NONE', #15959, #7096, #1943, .T. ) ;
#8190=PLANE ( 'NONE',  #4956 ) ;
#8226=FILL_AREA_STYLE ('',( #10417 ) ) ;
#8269=EDGE_LOOP ( 'NONE', ( #10486, #22728, #10878, #14473 ) ) ;
#8277=AXIS2_PLACEMENT_3D ( 'NONE', #20506, #5902, #6150 ) ;
#8357=EDGE_CURVE ( 'NONE', #19560, #21767, #21371, .T. ) ;
#8364=VERTEX_POINT ( 'NONE', #23296 ) ;
#8366=ADVANCED_FACE ( 'NONE', ( #4832 ), #14290, .T. ) ;
#8381=DIRECTION ( 'NONE',  ( 2.238759164535664589E-46, 3.469446951953614189E-15, 1.000000000000000000 ) ) ;
#8406=DIRECTION ( 'NONE',  ( 0.000000000000000000, 1.000000000000000000, 0.000000000000000000 ) ) ;
#8426=CARTESIAN_POINT ( 'NONE',  ( 65.00000000000004263, -52.79999999999959925, 65.00000000000018474 ) ) ;
#8438=AXIS2_PLACEMENT_3D ( 'NONE', #13273, #7677, #447 ) ;
#8452=DIRECTION ( 'NONE',  ( 4.625929269271484928E-16, -3.469446951953613794E-15, -1.000000000000000000 ) ) ;
#8463=CARTESIAN_POINT ( 'NONE',  ( 0.000000000000000000, 0.000000000000000000, -50.00000000000000000 ) ) ;
#8487=CARTESIAN_POINT ( 'NONE',  ( -44.99999999999997868, -56.79999999999937899, 140.0000000000001421 ) ) ;
#8488=( NAMED_UNIT ( * ) SI_UNIT ( $, .STERADIAN. ) SOLID_ANGLE_UNIT ( ) );
#8527=CARTESIAN_POINT ( 'NONE',  ( 25.00000000000001421, -37.41657386773940885, 169.9999999999999716 ) ) ;
#8546=CARTESIAN_POINT ( 'NONE',  ( 1.500000000000000000, 12.00000000000000000, 0.000000000000000000 ) ) ;
#8563=ORIENTED_EDGE ( 'NONE', *, *, #8189, .T. ) ;
#8574=VERTEX_POINT ( 'NONE', #7362 ) ;
#8590=DIRECTION ( 'NONE',  ( -1.000000000000000000, -3.736327486719275871E-16, -0.000000000000000000 ) ) ;
#8596=ORIENTED_EDGE ( 'NONE', *, *, #16136, .T. ) ;
#8603=CARTESIAN_POINT ( 'NONE',  ( 45.00000000000004974, -56.79999999999967031, 50.00000000000019895 ) ) ;
#8616=PLANE ( 'NONE',  #7309 ) ;
#8638=DIRECTION ( 'NONE',  ( -1.000000000000000000, 0.000000000000000000, 0.000000000000000000 ) ) ;
#8647=CARTESIAN_POINT ( 'NONE',  ( -44.99999999999995026, -56.79999999999969873, 50.00000000000019895 ) ) ;
#8692=VERTEX_POINT ( 'NONE', #22672 ) ;
#8704=EDGE_LOOP ( 'NONE', ( #19337, #13827, #3744, #1489 ) ) ;
#8726=DIRECTION ( 'NONE',  ( 0.000000000000000000, -3.469446951953614583E-15, -1.000000000000000000 ) ) ;
#8756=VECTOR ( 'NONE', #8590, 1000.000000000000000 ) ;
#8832=VERTEX_POINT ( 'NONE', #6738 ) ;
#8868=DIRECTION ( 'NONE',  ( -1.000000000000000000, 0.000000000000000000, 0.000000000000000000 ) ) ;
#8895=ORIENTED_EDGE ( 'NONE', *, *, #2658, .F. ) ;
#8931=ORIENTED_EDGE ( 'NONE', *, *, #7230, .T. ) ;
#8944=CARTESIAN_POINT ( 'NONE',  ( 0.000000000000000000, 0.000000000000000000, 169.9999999999999716 ) ) ;
#8955=( NAMED_UNIT ( * ) SI_UNIT ( $, .STERADIAN. ) SOLID_ANGLE_UNIT ( ) );
#8968=ORIENTED_EDGE ( 'NONE', *, *, #1443, .T. ) ;
#8997=LINE ( 'NONE', #1839, #20031 ) ;
#9025=DIRECTION ( 'NONE',  ( -3.736327486719275871E-16, 1.000000000000000000, 0.000000000000000000 ) ) ;
#9034=PRODUCT_DEFINITION_SHAPE ( 'NONE', 'NONE',  #12164 ) ;
#9037=AXIS2_PLACEMENT_3D ( 'NONE', #7080, #19993, #10618 ) ;
#9069=ORIENTED_EDGE ( 'NONE', *, *, #12569, .T. ) ;
#9081=LINE ( 'NONE', #16440, #18099 ) ;
#9130=DIRECTION ( 'NONE',  ( 0.000000000000000000, 0.000000000000000000, 1.000000000000000000 ) ) ;
#9134=ORIENTED_EDGE ( 'NONE', *, *, #5322, .F. ) ;
#9144=DIRECTION ( 'NONE',  ( -0.000000000000000000, -0.000000000000000000, -1.000000000000000000 ) ) ;
#9173=LINE ( 'NONE', #475, #3427 ) ;
#9184=LINE ( 'NONE', #12846, #23327 ) ;
#9227=DIRECTION ( 'NONE',  ( 3.736327486719275871E-16, -1.000000000000000000, 3.469446951953614189E-15 ) ) ;
#9291=PLANE ( 'NONE',  #23605 ) ;
#9314=ORIENTED_EDGE ( 'NONE', *, *, #12434, .F. ) ;
#9353=CARTESIAN_POINT ( 'NONE',  ( -64.99999999999997158, -52.79999999999974847, 35.00000000000017764 ) ) ;
#9358=DIRECTION ( 'NONE',  ( 0.000000000000000000, 0.000000000000000000, 1.000000000000000000 ) ) ;
#9373=VERTEX_POINT ( 'NONE', #3773 ) ;
#9380=DIRECTION ( 'NONE',  ( 0.000000000000000000, -3.469446951953614583E-15, -1.000000000000000000 ) ) ;
#9473=CARTESIAN_POINT ( 'NONE',  ( 0.000000000000000000, 0.000000000000000000, 0.000000000000000000 ) ) ;
#9490=DIRECTION ( 'NONE',  ( 1.000000000000000000, 0.000000000000000000, 0.000000000000000000 ) ) ;
#9565=ORIENTED_EDGE ( 'NONE', *, *, #585, .T. ) ;
#9569=DIRECTION ( 'NONE',  ( 0.000000000000000000, 2.618450529776326854E-15, 1.000000000000000000 ) ) ;
#9622=EDGE_CURVE ( 'NONE', #1592, #21376, #23088, .T. ) ;
#9634=CARTESIAN_POINT ( 'NONE',  ( 10.00000000000000000, 0.000000000000000000, -50.00000000000000000 ) ) ;
#9637=ORIENTED_EDGE ( 'NONE', *, *, #6978, .T. ) ;
#9642=VECTOR ( 'NONE', #1228, 1000.000000000000000 ) ;
#9644=VECTOR ( 'NONE', #300, 1000.000000000000000 ) ;
#9658=LINE ( 'NONE', #22664, #1094 ) ;
#9678=DIRECTION ( 'NONE',  ( 0.000000000000000000, 0.000000000000000000, 1.000000000000000000 ) ) ;
#9686=CARTESIAN_POINT ( 'NONE',  ( 1.983456134378398743E-14, -52.79999999999986215, 1.831306136874101694E-13 ) ) ;
#9708=DIRECTION ( 'NONE',  ( 0.000000000000000000, 2.618450529776326854E-15, 1.000000000000000000 ) ) ;
#9719=EDGE_CURVE ( 'NONE', #52, #17333, #20071, .T. ) ;
#9737=ORIENTED_EDGE ( 'NONE', *, *, #11263, .T. ) ;
#9741=DIRECTION ( 'NONE',  ( -2.238759164535664589E-46, -3.469446951953614189E-15, -1.000000000000000000 ) ) ;
#9782=ORIENTED_EDGE ( 'NONE', *, *, #22707, .T. ) ;
#9908=CARTESIAN_POINT ( 'NONE',  ( 1.500000000000000000, 0.000000000000000000, -50.00000000000000000 ) ) ;
#9926=ADVANCED_FACE ( 'NONE', ( #6855 ), #1417, .T. ) ;
#9956=VERTEX_POINT ( 'NONE', #12580 ) ;
#9977=CARTESIAN_POINT ( 'NONE',  ( -64.99999999999998579, -52.79999999999942872, 125.0000000000001421 ) ) ;
#10040=DIRECTION ( 'NONE',  ( 0.000000000000000000, 0.000000000000000000, 1.000000000000000000 ) ) ;
#10042=DIRECTION ( 'NONE',  ( 4.625929269271474081E-16, 0.000000000000000000, -1.000000000000000000 ) ) ;
#10114=CARTESIAN_POINT ( 'NONE',  ( 45.00000000000004974, -56.79999999999967741, 47.35000000000020037 ) ) ;
#10155=CARTESIAN_POINT ( 'NONE',  ( 65.00000000000004263, -52.79999999999959925, 65.00000000000018474 ) ) ;
#10166=VERTEX_POINT ( 'NONE', #1759 ) ;
#10169=ORIENTED_EDGE ( 'NONE', *, *, #5322, .T. ) ;
#10177=CARTESIAN_POINT ( 'NONE',  ( -25.00000000000001776, 45.00100000000062295, 124.9999999999998579 ) ) ;
#10198=PLANE ( 'NONE',  #5753 ) ;
#10226=EDGE_CURVE ( 'NONE', #4142, #13580, #23474, .T. ) ;
#10235=ADVANCED_FACE ( 'NONE', ( #21083 ), #5995, .T. ) ;
#10236=LINE ( 'NONE', #22783, #5205 ) ;
#10237=AXIS2_PLACEMENT_3D ( 'NONE', #10177, #17521, #12391 ) ;
#10258=VERTEX_POINT ( 'NONE', #17361 ) ;
#10272=VECTOR ( 'NONE', #23697, 1000.000000000000000 ) ;
#10287=VERTEX_POINT ( 'NONE', #15558 ) ;
#10302=VECTOR ( 'NONE', #1081, 1000.000000000000000 ) ;
#10321=FACE_BOUND ( 'NONE', #18423, .T. ) ;
#10399=DIRECTION ( 'NONE',  ( 0.000000000000000000, 0.000000000000000000, -1.000000000000000000 ) ) ;
#10411=EDGE_CURVE ( 'NONE', #11870, #3113, #12440, .T. ) ;
#10414=FACE_OUTER_BOUND ( 'NONE', #3578, .T. ) ;
#10417=FILL_AREA_STYLE_COLOUR ( '', #21165 ) ;
#10433=CIRCLE ( 'NONE', #4226, 2.649999999999992806 ) ;
#10440=CARTESIAN_POINT ( 'NONE',  ( 45.00000000000000711, 5.510910596163090344E-15, 169.9999999999999716 ) ) ;
#10455=CARTESIAN_POINT ( 'NONE',  ( 0.000000000000000000, 0.000000000000000000, -50.00000000000000000 ) ) ;
#10486=ORIENTED_EDGE ( 'NONE', *, *, #19677, .T. ) ;
#10554=LINE ( 'NONE', #4850, #5017 ) ;
#10618=DIRECTION ( 'NONE',  ( 0.000000000000000000, 2.618450529776326854E-15, 1.000000000000000000 ) ) ;
#10653=FACE_BOUND ( 'NONE', #1353, .T. ) ;
#10664=PLANE ( 'NONE',  #4058 ) ;
#10669=EDGE_LOOP ( 'NONE', ( #19915, #22319, #6548, #13891 ) ) ;
#10676=DIRECTION ( 'NONE',  ( 3.202566417187928841E-16, -1.000000000000000000, 3.469446951953614583E-15 ) ) ;
#10677=ADVANCED_FACE ( 'NONE', ( #21174 ), #8616, .F. ) ;
#10690=DIRECTION ( 'NONE',  ( -0.000000000000000000, 1.000000000000000000, -3.469446951953613794E-15 ) ) ;
#10696=FACE_BOUND ( 'NONE', #1061, .T. ) ;
#10739=AXIS2_PLACEMENT_3D ( 'NONE', #18104, #12589, #21827 ) ;
#10748=LINE ( 'NONE', #5414, #296 ) ;
#10774=PRESENTATION_STYLE_ASSIGNMENT (( #3495 ) ) ;
#10781=FACE_OUTER_BOUND ( 'NONE', #23305, .T. ) ;
#10784=EDGE_LOOP ( 'NONE', ( #14748, #17992, #591, #6964 ) ) ;
#10787=STYLED_ITEM ( 'NONE', ( #10774 ), #22256 ) ;
#10795=AXIS2_PLACEMENT_3D ( 'NONE', #17796, #10690, #1239 ) ;
#10830=VECTOR ( 'NONE', #20893, 1000.000000000000000 ) ;
#10838=CARTESIAN_POINT ( 'NONE',  ( 1.500000000000000000, 12.00000000000000000, -50.00000000000000000 ) ) ;
#10875=ORIENTED_EDGE ( 'NONE', *, *, #17351, .T. ) ;
#10878=ORIENTED_EDGE ( 'NONE', *, *, #2920, .F. ) ;
#10887=FACE_OUTER_BOUND ( 'NONE', #15008, .T. ) ;
#10888=ORIENTED_EDGE ( 'NONE', *, *, #14712, .F. ) ;
#10904=DIRECTION ( 'NONE',  ( 3.469446951953614682E-16, -1.000000000000000000, 3.483493295888648978E-15 ) ) ;
#10907=ORIENTED_EDGE ( 'NONE', *, *, #19759, .T. ) ;
#10908=DIRECTION ( 'NONE',  ( 2.238759164535664589E-46, 3.469446951953614189E-15, 1.000000000000000000 ) ) ;
#10933=EDGE_CURVE ( 'NONE', #13544, #15472, #16194, .T. ) ;
#10938=ORIENTED_EDGE ( 'NONE', *, *, #23482, .F. ) ;
#10945=EDGE_CURVE ( 'NONE', #1156, #7096, #14813, .T. ) ;
#11010=CARTESIAN_POINT ( 'NONE',  ( 45.00000000000002132, -52.79999999999936477, 140.0000000000001990 ) ) ;
#11018=LINE ( 'NONE', #3719, #22911 ) ;
#11042=CARTESIAN_POINT ( 'NONE',  ( -64.99999999999998579, -56.79999999999943583, 125.0000000000001705 ) ) ;
#11043=CARTESIAN_POINT ( 'NONE',  ( 0.000000000000000000, 0.000000000000000000, -50.00000000000000000 ) ) ;
#11109=DIRECTION ( 'NONE',  ( 0.000000000000000000, -2.618450529776326854E-15, -1.000000000000000000 ) ) ;
#11152=CIRCLE ( 'NONE', #11944, 2.649999999999985700 ) ;
#11178=LINE ( 'NONE', #16702, #16937 ) ;
#11208=LINE ( 'NONE', #14925, #19916 ) ;
#11210=AXIS2_PLACEMENT_3D ( 'NONE', #9473, #14914, #3769 ) ;
#11226=EDGE_CURVE ( 'NONE', #5058, #4246, #14854, .T. ) ;
#11263=EDGE_CURVE ( 'NONE', #436, #1277, #21416, .T. ) ;
#11284=DIRECTION ( 'NONE',  ( -0.000000000000000000, 1.000000000000000000, -3.469446951953613794E-15 ) ) ;
#11287=ORIENTED_EDGE ( 'NONE', *, *, #13790, .F. ) ;
#11334=DIRECTION ( 'NONE',  ( 0.000000000000000000, 0.000000000000000000, 1.000000000000000000 ) ) ;
#11337=ORIENTED_EDGE ( 'NONE', *, *, #19808, .F. ) ;
#11361=ORIENTED_EDGE ( 'NONE', *, *, #5192, .F. ) ;
#11370=CYLINDRICAL_SURFACE ( 'NONE', #8277, 2.649999999999985700 ) ;
#11408=CARTESIAN_POINT ( 'NONE',  ( -45.00000000000000711, 0.000000000000000000, 169.9999999999999716 ) ) ;
#11451=DIRECTION ( 'NONE',  ( -1.000000000000000000, -3.202566417187951028E-16, -6.405132834375902056E-16 ) ) ;
#11472=VECTOR ( 'NONE', #1813, 1000.000000000000000 ) ;
#11544=ORIENTED_EDGE ( 'NONE', *, *, #13943, .T. ) ;
#11568=( GEOMETRIC_REPRESENTATION_CONTEXT ( 3 ) GLOBAL_UNCERTAINTY_ASSIGNED_CONTEXT ( ( #14745 ) ) GLOBAL_UNIT_ASSIGNED_CONTEXT ( ( #20585, #7011, #8955 ) ) REPRESENTATION_CONTEXT ( 'NONE', 'WORKASPACE' ) );
#11592=ADVANCED_FACE ( 'NONE', ( #13802 ), #17399, .T. ) ;
#11599=CIRCLE ( 'NONE', #7695, 45.00000000000000711 ) ;
#11600=VECTOR ( 'NONE', #324, 1000.000000000000000 ) ;
#11623=ORIENTED_EDGE ( 'NONE', *, *, #10933, .F. ) ;
#11624=EDGE_CURVE ( 'NONE', #3113, #22598, #14034, .T. ) ;
#11635=FACE_OUTER_BOUND ( 'NONE', #16033, .T. ) ;
#11642=FACE_BOUND ( 'NONE', #21865, .T. ) ;
#11655=ORIENTED_EDGE ( 'NONE', *, *, #9719, .F. ) ;
#11663=EDGE_CURVE ( 'NONE', #23309, #15457, #21828, .T. ) ;
#11690=CARTESIAN_POINT ( 'NONE',  ( 0.000000000000000000, 0.000000000000000000, 125.0000000000000284 ) ) ;
#11752=ORIENTED_EDGE ( 'NONE', *, *, #5098, .F. ) ;
#11787=ORIENTED_EDGE ( 'NONE', *, *, #13943, .F. ) ;
#11817=LINE ( 'NONE', #10440, #9642 ) ;
#11832=ORIENTED_EDGE ( 'NONE', *, *, #21176, .T. ) ;
#11865=EDGE_CURVE ( 'NONE', #21387, #21376, #22887, .T. ) ;
#11866=CARTESIAN_POINT ( 'NONE',  ( -25.00000000000001776, 45.00100000000062295, 124.9999999999998579 ) ) ;
#11869=PLANE ( 'NONE',  #4442 ) ;
#11870=VERTEX_POINT ( 'NONE', #13060 ) ;
#11944=AXIS2_PLACEMENT_3D ( 'NONE', #11010, #20609, #16531 ) ;
#11976=DIRECTION ( 'NONE',  ( 0.000000000000000000, 2.618450529776319755E-15, 1.000000000000000000 ) ) ;
#11978=DIRECTION ( 'NONE',  ( -1.000000000000000000, -3.469446951953598905E-16, 4.625929269271498733E-16 ) ) ;
#12006=ORIENTED_EDGE ( 'NONE', *, *, #11865, .T. ) ;
#12042=LINE ( 'NONE', #22727, #18825 ) ;
#12043=ORIENTED_EDGE ( 'NONE', *, *, #17351, .F. ) ;
#12053=DIRECTION ( 'NONE',  ( 0.000000000000000000, 0.000000000000000000, 1.000000000000000000 ) ) ;
#12092=CARTESIAN_POINT ( 'NONE',  ( 25.00000000000004263, -37.41657386773938754, 35.00000000000013500 ) ) ;
#12096=DIRECTION ( 'NONE',  ( 0.000000000000000000, 1.000000000000000000, 0.000000000000000000 ) ) ;
#12164=PRODUCT_DEFINITION ( 'UNKNOWN', '', #2322, #1789 ) ;
#12210=DIRECTION ( 'NONE',  ( -4.625929269271485914E-16, 3.469446951953614583E-15, 1.000000000000000000 ) ) ;
#12230=LINE ( 'NONE', #10155, #21415 ) ;
#12254=PLANE ( 'NONE',  #10237 ) ;
#12262=PLANE ( 'NONE',  #8088 ) ;
#12272=FACE_OUTER_BOUND ( 'NONE', #19847, .T. ) ;
#12346=DIRECTION ( 'NONE',  ( 0.000000000000000000, -1.000000000000000000, 3.469446951953614189E-15 ) ) ;
#12349=CIRCLE ( 'NONE', #1863, 10.00000000000000000 ) ;
#12387=AXIS2_PLACEMENT_3D ( 'NONE', #21351, #2979, #12346 ) ;
#12388=VECTOR ( 'NONE', #14755, 1000.000000000000000 ) ;
#12391=DIRECTION ( 'NONE',  ( 0.000000000000000000, 1.000000000000000000, -3.469446951953614189E-15 ) ) ;
#12411=DIRECTION ( 'NONE',  ( 1.000000000000000000, 0.000000000000000000, -0.000000000000000000 ) ) ;
#12415=ORIENTED_EDGE ( 'NONE', *, *, #23452, .T. ) ;
#12418=FACE_OUTER_BOUND ( 'NONE', #13706, .T. ) ;
#12427=CARTESIAN_POINT ( 'NONE',  ( 25.00000000000004974, -52.79999999999962057, 65.00000000000018474 ) ) ;
#12434=EDGE_CURVE ( 'NONE', #8692, #1257, #3296, .T. ) ;
#12440=LINE ( 'NONE', #1270, #7286 ) ;
#12443=EDGE_CURVE ( 'NONE', #840, #2982, #16596, .T. ) ;
#12477=CARTESIAN_POINT ( 'NONE',  ( 24.99999999999998579, 45.00100000000064426, 124.9999999999998579 ) ) ;
#12485=VERTEX_POINT ( 'NONE', #4619 ) ;
#12495=AXIS2_PLACEMENT_3D ( 'NONE', #5434, #16310, #18567 ) ;
#12516=FACE_OUTER_BOUND ( 'NONE', #7131, .T. ) ;
#12517=CYLINDRICAL_SURFACE ( 'NONE', #14270, 10.00000000000000000 ) ;
#12564=DIRECTION ( 'NONE',  ( 3.736327486719275871E-16, -1.000000000000000000, 3.469446951953614189E-15 ) ) ;
#12569=EDGE_CURVE ( 'NONE', #9373, #18998, #22599, .T. ) ;
#12580=CARTESIAN_POINT ( 'NONE',  ( -1.500000000000000000, 9.886859966642592923, 0.000000000000000000 ) ) ;
#12587=VECTOR ( 'NONE', #19663, 1000.000000000000000 ) ;
#12588=VERTEX_POINT ( 'NONE', #19094 ) ;
#12589=DIRECTION ( 'NONE',  ( 3.202566417187928841E-16, -1.000000000000000000, 3.469446951953614583E-15 ) ) ;
#12598=CLOSED_SHELL ( 'NONE', ( #17007, #5232, #3310, #7430, #15561, #3365, #3847, #3334, #3374, #1376, #7227, #23333, #9926, #10235, #8366, #1800, #12767, #1155, #19324, #17744, #5196, #1218, #11592, #4254, #6612, #1379, #6094, #12987, #6896, #21104, #10677, #1905, #7172, #4467, #182, #17997, #6762 ) ) ;
#12608=MANIFOLD_SOLID_BREP ( 'M5 Clearance Hole1', #12598 ) ;
#12627=VERTEX_POINT ( 'NONE', #2899 ) ;
#12643=VERTEX_POINT ( 'NONE', #21640 ) ;
#12683=FACE_OUTER_BOUND ( 'NONE', #19281, .T. ) ;
#12699=DIRECTION ( 'NONE',  ( 3.736327486719275871E-16, -1.000000000000000000, 3.469446951953613794E-15 ) ) ;
#12709=DIRECTION ( 'NONE',  ( -0.000000000000000000, 1.000000000000000000, -3.469446951953613794E-15 ) ) ;
#12731=EDGE_CURVE ( 'NONE', #10287, #1156, #15355, .T. ) ;
#12766=FACE_OUTER_BOUND ( 'NONE', #4398, .T. ) ;
#12767=ADVANCED_FACE ( 'NONE', ( #6486 ), #21456, .F. ) ;
#12795=ORIENTED_EDGE ( 'NONE', *, *, #10933, .T. ) ;
#12842=DIRECTION ( 'NONE',  ( -0.000000000000000000, 1.000000000000000000, -3.469446951953613794E-15 ) ) ;
#12846=CARTESIAN_POINT ( 'NONE',  ( 25.00000000000001066, 45.00100000000033162, 34.99999999999983658 ) ) ;
#12847=DIRECTION ( 'NONE',  ( 0.000000000000000000, 2.618450529776313049E-15, 1.000000000000000000 ) ) ;
#12859=EDGE_CURVE ( 'NONE', #18998, #1257, #2464, .T. ) ;
#12872=ORIENTED_EDGE ( 'NONE', *, *, #20465, .T. ) ;
#12875=ORIENTED_EDGE ( 'NONE', *, *, #9719, .T. ) ;
#12906=VECTOR ( 'NONE', #5180, 1000.000000000000000 ) ;
#12917=CARTESIAN_POINT ( 'NONE',  ( 1.500000000000000000, 9.886859966642592923, -50.00000000000000000 ) ) ;
#12938=DIRECTION ( 'NONE',  ( 0.000000000000000000, -3.469446951953614583E-15, -1.000000000000000000 ) ) ;
#12952=AXIS2_PLACEMENT_3D ( 'NONE', #20595, #14836, #4312 ) ;
#12987=ADVANCED_FACE ( 'NONE', ( #18762, #20704 ), #22514, .F. ) ;
#13023=ORIENTED_EDGE ( 'NONE', *, *, #271, .F. ) ;
#13038=LINE ( 'NONE', #12917, #15399 ) ;
#13044=AXIS2_PLACEMENT_3D ( 'NONE', #15474, #2762, #15827 ) ;
#13053=FACE_BOUND ( 'NONE', #993, .T. ) ;
#13060=CARTESIAN_POINT ( 'NONE',  ( 1.500000000000000000, 9.886859966642592923, 0.000000000000000000 ) ) ;
#13088=CARTESIAN_POINT ( 'NONE',  ( 65.00000000000002842, -56.79999999999928662, 155.0000000000002558 ) ) ;
#13104=ORIENTED_EDGE ( 'NONE', *, *, #4552, .T. ) ;
#13205=DIRECTION ( 'NONE',  ( 0.000000000000000000, 1.000000000000000000, 0.000000000000000000 ) ) ;
#13212=ORIENTED_EDGE ( 'NONE', *, *, #15885, .F. ) ;
#13273=CARTESIAN_POINT ( 'NONE',  ( -1.500000000000000000, 0.000000000000000000, 0.000000000000000000 ) ) ;
#13294=VERTEX_POINT ( 'NONE', #21668 ) ;
#13301=DIRECTION ( 'NONE',  ( -0.000000000000000000, 1.000000000000000000, -3.469446951953613794E-15 ) ) ;
#13352=CIRCLE ( 'NONE', #6371, 2.649999999999985700 ) ;
#13353=DIRECTION ( 'NONE',  ( -3.736327486719275871E-16, 1.000000000000000000, 0.000000000000000000 ) ) ;
#13404=AXIS2_PLACEMENT_3D ( 'NONE', #1792, #3254, #12847 ) ;
#13453=VERTEX_POINT ( 'NONE', #9353 ) ;
#13470=DIRECTION ( 'NONE',  ( -0.000000000000000000, 1.000000000000000000, -3.469446951953613794E-15 ) ) ;
#13507=EDGE_CURVE ( 'NONE', #2833, #21387, #12042, .T. ) ;
#13517=ORIENTED_EDGE ( 'NONE', *, *, #23493, .F. ) ;
#13522=CARTESIAN_POINT ( 'NONE',  ( -24.99999999999996092, -37.41657386773943728, 65.00000000000012790 ) ) ;
#13544=VERTEX_POINT ( 'NONE', #20919 ) ;
#13564=CYLINDRICAL_SURFACE ( 'NONE', #22462, 2.649999999999999467 ) ;
#13580=VERTEX_POINT ( 'NONE', #13609 ) ;
#13609=CARTESIAN_POINT ( 'NONE',  ( -10.00000000000000000, 1.224646799147353256E-15, 20.00000000000000000 ) ) ;
#13629=EDGE_CURVE ( 'NONE', #12485, #18619, #7648, .T. ) ;
#13638=CARTESIAN_POINT ( 'NONE',  ( 0.000000000000000000, 0.000000000000000000, 65.00000000000000000 ) ) ;
#13645=EDGE_CURVE ( 'NONE', #1257, #18998, #15001, .T. ) ;
#13653=DIRECTION ( 'NONE',  ( 1.000000000000000000, 3.736327486719275871E-16, -1.296299001029869881E-30 ) ) ;
#13685=ORIENTED_EDGE ( 'NONE', *, *, #4902, .F. ) ;
#13706=EDGE_LOOP ( 'NONE', ( #20156, #22482, #19183, #14398 ) ) ;
#13714=PLANE ( 'NONE',  #6010 ) ;
#13718=AXIS2_PLACEMENT_3D ( 'NONE', #11690, #8381, #17917 ) ;
#13759=CIRCLE ( 'NONE', #16423, 10.00000000000000000 ) ;
#13790=EDGE_CURVE ( 'NONE', #18606, #23584, #22317, .T. ) ;
#13794=VERTEX_POINT ( 'NONE', #21643 ) ;
#13802=FACE_OUTER_BOUND ( 'NONE', #21344, .T. ) ;
#13827=ORIENTED_EDGE ( 'NONE', *, *, #17778, .F. ) ;
#13852=FACE_OUTER_BOUND ( 'NONE', #2244, .T. ) ;
#13860=CARTESIAN_POINT ( 'NONE',  ( 0.000000000000000000, 0.000000000000000000, 20.00000000000000000 ) ) ;
#13874=AXIS2_PLACEMENT_3D ( 'NONE', #8603, #7026, #14307 ) ;
#13891=ORIENTED_EDGE ( 'NONE', *, *, #11226, .F. ) ;
#13900=CARTESIAN_POINT ( 'NONE',  ( -1.500000000000000000, 0.000000000000000000, -50.00000000000000000 ) ) ;
#13909=ORIENTED_EDGE ( 'NONE', *, *, #19227, .T. ) ;
#13927=DIRECTION ( 'NONE',  ( 3.469446951953614682E-16, -1.000000000000000000, 3.483493295888648978E-15 ) ) ;
#13943=EDGE_CURVE ( 'NONE', #12485, #19969, #9081, .T. ) ;
#13948=CIRCLE ( 'NONE', #4650, 2.649999999999992806 ) ;
#13971=DIRECTION ( 'NONE',  ( -0.000000000000000000, 1.000000000000000000, -3.469446951953613794E-15 ) ) ;
#13976=ORIENTED_EDGE ( 'NONE', *, *, #5514, .T. ) ;
#13977=CARTESIAN_POINT ( 'NONE',  ( 2.122234012456543311E-14, -56.79999999999985505, 1.970645868709647558E-13 ) ) ;
#14017=ORIENTED_EDGE ( 'NONE', *, *, #5514, .F. ) ;
#14034=LINE ( 'NONE', #2991, #3986 ) ;
#14041=DIRECTION ( 'NONE',  ( 1.000000000000000000, 0.000000000000000000, 0.000000000000000000 ) ) ;
#14067=DIRECTION ( 'NONE',  ( 1.000000000000000000, 0.000000000000000000, 0.000000000000000000 ) ) ;
#14091=ORIENTED_EDGE ( 'NONE', *, *, #21561, .T. ) ;
#14122=LINE ( 'NONE', #6973, #21909 ) ;
#14149=CARTESIAN_POINT ( 'NONE',  ( 24.99999999999998579, 45.00100000000064426, 124.9999999999998579 ) ) ;
#14159=PLANE ( 'NONE',  #20529 ) ;
#14200=ORIENTED_EDGE ( 'NONE', *, *, #1639, .F. ) ;
#14264=EDGE_LOOP ( 'NONE', ( #21419, #12415, #5463, #13685 ) ) ;
#14270=AXIS2_PLACEMENT_3D ( 'NONE', #10455, #12053, #5109 ) ;
#14290=PLANE ( 'NONE',  #17248 ) ;
#14297=CARTESIAN_POINT ( 'NONE',  ( -64.99999999999995737, -52.79999999999965610, 65.00000000000017053 ) ) ;
#14307=DIRECTION ( 'NONE',  ( 0.000000000000000000, -2.618450529776313049E-15, -1.000000000000000000 ) ) ;
#14321=CYLINDRICAL_SURFACE ( 'NONE', #10795, 2.649999999999985700 ) ;
#14347=ORIENTED_EDGE ( 'NONE', *, *, #22341, .F. ) ;
#14373=EDGE_LOOP ( 'NONE', ( #17670, #16236, #7496, #4874 ) ) ;
#14380=ORIENTED_EDGE ( 'NONE', *, *, #21969, .T. ) ;
#14398=ORIENTED_EDGE ( 'NONE', *, *, #3538, .T. ) ;
#14456=AXIS2_PLACEMENT_3D ( 'NONE', #16173, #12699, #21711 ) ;
#14473=ORIENTED_EDGE ( 'NONE', *, *, #4495, .T. ) ;
#14475=CARTESIAN_POINT ( 'NONE',  ( -64.99999999999998579, -56.79999999999943583, 125.0000000000001705 ) ) ;
#14564=CIRCLE ( 'NONE', #10739, 2.649999999999985700 ) ;
#14569=CARTESIAN_POINT ( 'NONE',  ( 0.000000000000000000, 0.000000000000000000, -50.00000000000000000 ) ) ;
#14612=LINE ( 'NONE', #3592, #2016 ) ;
#14618=AXIS2_PLACEMENT_3D ( 'NONE', #21158, #15513, #15271 ) ;
#14641=LINE ( 'NONE', #19697, #22290 ) ;
#14712=EDGE_CURVE ( 'NONE', #15457, #52, #16390, .T. ) ;
#14730=CARTESIAN_POINT ( 'NONE',  ( 45.00000000000002132, -56.79999999999934346, 142.6500000000002046 ) ) ;
#14731=CARTESIAN_POINT ( 'NONE',  ( 65.00000000000001421, -52.79999999999938609, 125.0000000000002274 ) ) ;
#14739=LINE ( 'NONE', #1673, #23240 ) ;
#14745=UNCERTAINTY_MEASURE_WITH_UNIT (LENGTH_MEASURE( 1.000000000000000082E-05 ), #20585, 'distance_accuracy_value', 'NONE');
#14748=ORIENTED_EDGE ( 'NONE', *, *, #13790, .T. ) ;
#14755=DIRECTION ( 'NONE',  ( 4.625929269271486900E-16, 3.469446951953614978E-15, 1.000000000000000000 ) ) ;
#14783=ORIENTED_EDGE ( 'NONE', *, *, #3963, .F. ) ;
#14801=VECTOR ( 'NONE', #8638, 1000.000000000000000 ) ;
#14813=LINE ( 'NONE', #16842, #9644 ) ;
#14816=AXIS2_PLACEMENT_3D ( 'NONE', #8426, #4797, #15236 ) ;
#14836=DIRECTION ( 'NONE',  ( 0.000000000000000000, 0.000000000000000000, 1.000000000000000000 ) ) ;
#14844=EDGE_CURVE ( 'NONE', #13544, #4142, #7924, .T. ) ;
#14854=CIRCLE ( 'NONE', #13718, 45.00000000000000711 ) ;
#14855=CARTESIAN_POINT ( 'NONE',  ( -64.99999999999995737, -52.79999999999965610, 65.00000000000017053 ) ) ;
#14860=EDGE_LOOP ( 'NONE', ( #19089, #4382, #18052, #5241 ) ) ;
#14874=CARTESIAN_POINT ( 'NONE',  ( -64.99999999999995737, -52.79999999999965610, 65.00000000000017053 ) ) ;
#14886=CIRCLE ( 'NONE', #21762, 45.00000000000000711 ) ;
#14895=ORIENTED_EDGE ( 'NONE', *, *, #10411, .T. ) ;
#14914=DIRECTION ( 'NONE',  ( 0.000000000000000000, 0.000000000000000000, 1.000000000000000000 ) ) ;
#14920=VERTEX_POINT ( 'NONE', #2366 ) ;
#14925=CARTESIAN_POINT ( 'NONE',  ( -64.99999999999998579, -52.79999999999942872, 125.0000000000001421 ) ) ;
#14950=VECTOR ( 'NONE', #10040, 1000.000000000000000 ) ;
#14966=CARTESIAN_POINT ( 'NONE',  ( 45.00000000000002132, -52.79999999999936477, 140.0000000000001990 ) ) ;
#14976=EDGE_CURVE ( 'NONE', #13294, #3415, #4307, .T. ) ;
#15001=CIRCLE ( 'NONE', #20381, 2.649999999999985700 ) ;
#15008=EDGE_LOOP ( 'NONE', ( #10888, #1424, #2885, #11655 ) ) ;
#15026=DIRECTION ( 'NONE',  ( -1.000000000000000000, -3.736327486719275871E-16, -0.000000000000000000 ) ) ;
#15053=DIRECTION ( 'NONE',  ( 3.469446951953614682E-16, -1.000000000000000000, 3.483493295888648978E-15 ) ) ;
#15078=AXIS2_PLACEMENT_3D ( 'NONE', #4423, #13653, #15313 ) ;
#15079=ORIENTED_EDGE ( 'NONE', *, *, #8123, .T. ) ;
#15104=ORIENTED_EDGE ( 'NONE', *, *, #14976, .T. ) ;
#15123=DIRECTION ( 'NONE',  ( 0.000000000000000000, -3.469446951953613794E-15, -1.000000000000000000 ) ) ;
#15139=ORIENTED_EDGE ( 'NONE', *, *, #1940, .F. ) ;
#15147=CARTESIAN_POINT ( 'NONE',  ( -25.00000000000001776, 45.00100000000062295, 124.9999999999998579 ) ) ;
#15197=MECHANICAL_DESIGN_GEOMETRIC_PRESENTATION_REPRESENTATION('',(#7853),#17490);
#15236=DIRECTION ( 'NONE',  ( -4.625929269271472109E-16, 0.000000000000000000, 1.000000000000000000 ) ) ;
#15271=DIRECTION ( 'NONE',  ( 1.776356839400250465E-15, 1.000000000000000000, -3.546545773108138379E-15 ) ) ;
#15284=VECTOR ( 'NONE', #2522, 1000.000000000000000 ) ;
#15292=ORIENTED_EDGE ( 'NONE', *, *, #488, .F. ) ;
#15307=ORIENTED_EDGE ( 'NONE', *, *, #267, .T. ) ;
#15313=DIRECTION ( 'NONE',  ( -3.736327486719275871E-16, 1.000000000000000000, 0.000000000000000000 ) ) ;
#15314=CARTESIAN_POINT ( 'NONE',  ( -24.99999999999998224, -52.79999999999944293, 125.0000000000001990 ) ) ;
#15342=LINE ( 'NONE', #9908, #17963 ) ;
#15355=LINE ( 'NONE', #4227, #7870 ) ;
#15364=ORIENTED_EDGE ( 'NONE', *, *, #12569, .F. ) ;
#15399=VECTOR ( 'NONE', #16741, 1000.000000000000000 ) ;
#15457=VERTEX_POINT ( 'NONE', #15744 ) ;
#15458=DIRECTION ( 'NONE',  ( 4.625929269271484928E-16, -3.469446951953613794E-15, -1.000000000000000000 ) ) ;
#15472=VERTEX_POINT ( 'NONE', #15522 ) ;
#15474=CARTESIAN_POINT ( 'NONE',  ( 45.00000000000004974, -52.79999999999967031, 50.00000000000018474 ) ) ;
#15480=CARTESIAN_POINT ( 'NONE',  ( -44.99999999999995026, -56.79999999999970584, 47.35000000000020037 ) ) ;
#15513=DIRECTION ( 'NONE',  ( 2.238759164535664589E-46, 3.469446951953614189E-15, 1.000000000000000000 ) ) ;
#15515=CARTESIAN_POINT ( 'NONE',  ( 0.000000000000000000, 0.000000000000000000, 20.00000000000000000 ) ) ;
#15522=CARTESIAN_POINT ( 'NONE',  ( 1.500000000000000000, 9.886859966642592923, -50.00000000000000000 ) ) ;
#15546=PLANE ( 'NONE',  #8438 ) ;
#15558=CARTESIAN_POINT ( 'NONE',  ( -64.99999999999998579, -52.79999999999942872, 125.0000000000001421 ) ) ;
#15561=ADVANCED_FACE ( 'NONE', ( #12516 ), #18249, .T. ) ;
#15563=CARTESIAN_POINT ( 'NONE',  ( 1.500000000000000000, 12.00000000000000000, 0.000000000000000000 ) ) ;
#15564=CARTESIAN_POINT ( 'NONE',  ( 45.00000000000004974, -52.79999999999967741, 47.35000000000019327 ) ) ;
#15585=VECTOR ( 'NONE', #11284, 1000.000000000000000 ) ;
#15589=LINE ( 'NONE', #11866, #4903 ) ;
#15605=SURFACE_STYLE_FILL_AREA ( #8226 ) ;
#15678=ORIENTED_EDGE ( 'NONE', *, *, #9622, .F. ) ;
#15716=DIRECTION ( 'NONE',  ( 1.000000000000000000, 0.000000000000000000, 0.000000000000000000 ) ) ;
#15744=CARTESIAN_POINT ( 'NONE',  ( 65.00000000000001421, -56.79999999999939320, 125.0000000000002558 ) ) ;
#15800=ORIENTED_EDGE ( 'NONE', *, *, #5579, .T. ) ;
#15804=VECTOR ( 'NONE', #7764, 1000.000000000000000 ) ;
#15812=VECTOR ( 'NONE', #3589, 1000.000000000000000 ) ;
#15827=DIRECTION ( 'NONE',  ( 0.000000000000000000, 2.618450529776319755E-15, 1.000000000000000000 ) ) ;
#15844=CARTESIAN_POINT ( 'NONE',  ( -65.00000000000000000, -56.79999999999932925, 155.0000000000001705 ) ) ;
#15845=DIRECTION ( 'NONE',  ( 0.000000000000000000, 0.000000000000000000, 1.000000000000000000 ) ) ;
#15857=DIRECTION ( 'NONE',  ( -4.625929269271499719E-16, 0.000000000000000000, -1.000000000000000000 ) ) ;
#15885=EDGE_CURVE ( 'NONE', #22598, #10166, #10748, .T. ) ;
#15951=CARTESIAN_POINT ( 'NONE',  ( 0.000000000000000000, 0.000000000000000000, 20.00000000000000000 ) ) ;
#15957=CIRCLE ( 'NONE', #1662, 10.00000000000000000 ) ;
#15959=VERTEX_POINT ( 'NONE', #15314 ) ;
#16033=EDGE_LOOP ( 'NONE', ( #12875, #22450, #7981, #6099 ) ) ;
#16090=CARTESIAN_POINT ( 'NONE',  ( 1.680279846884594175E-14, -52.79999999999984794, 1.831306136874101946E-13 ) ) ;
#16106=FACE_BOUND ( 'NONE', #3724, .T. ) ;
#16136=EDGE_CURVE ( 'NONE', #21370, #4511, #3007, .T. ) ;
#16155=PLANE ( 'NONE',  #4972 ) ;
#16173=CARTESIAN_POINT ( 'NONE',  ( -44.99999999999995026, -56.79999999999969873, 50.00000000000019895 ) ) ;
#16180=ORIENTED_EDGE ( 'NONE', *, *, #2920, .T. ) ;
#16194=CIRCLE ( 'NONE', #18116, 10.00000000000000000 ) ;
#16203=CYLINDRICAL_SURFACE ( 'NONE', #13404, 2.649999999999999467 ) ;
#16236=ORIENTED_EDGE ( 'NONE', *, *, #4761, .T. ) ;
#16285=VERTEX_POINT ( 'NONE', #1849 ) ;
#16298=LINE ( 'NONE', #23642, #23320 ) ;
#16303=ORIENTED_EDGE ( 'NONE', *, *, #713, .F. ) ;
#16310=DIRECTION ( 'NONE',  ( 3.202566417187928841E-16, -1.000000000000000000, 3.469446951953614583E-15 ) ) ;
#16329=CARTESIAN_POINT ( 'NONE',  ( -44.99999999999995026, -52.79999999999969873, 50.00000000000018474 ) ) ;
#16348=LINE ( 'NONE', #18506, #10272 ) ;
#16350=DIRECTION ( 'NONE',  ( -0.000000000000000000, 1.000000000000000000, -3.469446951953613794E-15 ) ) ;
#16353=AXIS2_PLACEMENT_3D ( 'NONE', #14149, #21125, #19308 ) ;
#16390=LINE ( 'NONE', #14475, #5793 ) ;
#16423=AXIS2_PLACEMENT_3D ( 'NONE', #13860, #20944, #3294 ) ;
#16440=CARTESIAN_POINT ( 'NONE',  ( -24.99999999999996092, -37.41657386773943728, 169.9999999999999716 ) ) ;
#16481=DIRECTION ( 'NONE',  ( 0.000000000000000000, 0.000000000000000000, 1.000000000000000000 ) ) ;
#16489=ORIENTED_EDGE ( 'NONE', *, *, #1940, .T. ) ;
#16510=ORIENTED_EDGE ( 'NONE', *, *, #3928, .T. ) ;
#16531=DIRECTION ( 'NONE',  ( 0.000000000000000000, 2.618450529776326854E-15, 1.000000000000000000 ) ) ;
#16534=CIRCLE ( 'NONE', #16908, 2.649999999999992806 ) ;
#16543=DIRECTION ( 'NONE',  ( 3.736327486719275871E-16, -1.000000000000000000, 3.469446951953614189E-15 ) ) ;
#16596=LINE ( 'NONE', #5708, #20953 ) ;
#16621=ORIENTED_EDGE ( 'NONE', *, *, #4552, .F. ) ;
#16671=AXIS2_PLACEMENT_3D ( 'NONE', #21625, #6647, #14041 ) ;
#16675=ORIENTED_EDGE ( 'NONE', *, *, #7698, .F. ) ;
#16678=DIRECTION ( 'NONE',  ( -0.000000000000000000, 3.469446951953613794E-15, 1.000000000000000000 ) ) ;
#16702=CARTESIAN_POINT ( 'NONE',  ( 25.00000000000004974, -52.79999999999973426, 35.00000000000017764 ) ) ;
#16726=CARTESIAN_POINT ( 'NONE',  ( -10.00000000000000000, 1.224646799147353256E-15, -50.00000000000000000 ) ) ;
#16741=DIRECTION ( 'NONE',  ( 0.000000000000000000, 0.000000000000000000, 1.000000000000000000 ) ) ;
#16775=APPLICATION_CONTEXT ( 'automotive_design' ) ;
#16782=AXIS2_PLACEMENT_3D ( 'NONE', #8944, #3789, #5975 ) ;
#16829=ORIENTED_EDGE ( 'NONE', *, *, #12859, .T. ) ;
#16842=CARTESIAN_POINT ( 'NONE',  ( -65.00000000000000000, -52.79999999999933635, 155.0000000000001421 ) ) ;
#16851=CARTESIAN_POINT ( 'NONE',  ( 1.680279846884594175E-14, -52.79999999999984794, 1.831306136874101946E-13 ) ) ;
#16859=CARTESIAN_POINT ( 'NONE',  ( -64.99999999999995737, -56.79999999999964899, 65.00000000000018474 ) ) ;
#16869=LINE ( 'NONE', #23754, #486 ) ;
#16908=AXIS2_PLACEMENT_3D ( 'NONE', #23013, #6483, #11976 ) ;
#16929=EDGE_CURVE ( 'NONE', #6553, #13453, #4605, .T. ) ;
#16937=VECTOR ( 'NONE', #51, 1000.000000000000000 ) ;
#16981=ORIENTED_EDGE ( 'NONE', *, *, #3928, .F. ) ;
#17007=ADVANCED_FACE ( 'NONE', ( #10781 ), #16203, .F. ) ;
#17032=CARTESIAN_POINT ( 'NONE',  ( -64.99999999999998579, -52.79999999999942872, 125.0000000000001421 ) ) ;
#17085=ORIENTED_EDGE ( 'NONE', *, *, #19631, .F. ) ;
#17146=ORIENTED_EDGE ( 'NONE', *, *, #19768, .F. ) ;
#17162=AXIS2_PLACEMENT_3D ( 'NONE', #17032, #6026, #10042 ) ;
#17201=EDGE_CURVE ( 'NONE', #14920, #436, #18686, .T. ) ;
#17202=ORIENTED_EDGE ( 'NONE', *, *, #5192, .T. ) ;
#17239=CARTESIAN_POINT ( 'NONE',  ( -24.99999999999998224, -52.79999999999934346, 155.0000000000001990 ) ) ;
#17248=AXIS2_PLACEMENT_3D ( 'NONE', #3247, #6650, #6526 ) ;
#17311=EDGE_CURVE ( 'NONE', #7027, #21871, #23779, .T. ) ;
#17333=VERTEX_POINT ( 'NONE', #4458 ) ;
#17343=ORIENTED_EDGE ( 'NONE', *, *, #11226, .T. ) ;
#17351=EDGE_CURVE ( 'NONE', #5058, #15959, #15589, .T. ) ;
#17353=EDGE_CURVE ( 'NONE', #5058, #19016, #19174, .T. ) ;
#17361=CARTESIAN_POINT ( 'NONE',  ( -1.500000000000000000, 9.886859966642592923, -50.00000000000000000 ) ) ;
#17399=PLANE ( 'NONE',  #16353 ) ;
#17478=EDGE_LOOP ( 'NONE', ( #731, #3324, #23252, #13104 ) ) ;
#17490=( GEOMETRIC_REPRESENTATION_CONTEXT ( 3 ) GLOBAL_UNCERTAINTY_ASSIGNED_CONTEXT ( ( #753 ) ) GLOBAL_UNIT_ASSIGNED_CONTEXT ( ( #23433, #6550, #8488 ) ) REPRESENTATION_CONTEXT ( 'NONE', 'WORKASPACE' ) );
#17497=CARTESIAN_POINT ( 'NONE',  ( 65.00000000000002842, -52.79999999999929372, 155.0000000000002274 ) ) ;
#17508=EDGE_LOOP ( 'NONE', ( #14783, #15307, #20812, #19687, #9637, #9782, #3528, #17530 ) ) ;
#17521=DIRECTION ( 'NONE',  ( -2.238759164535664589E-46, -3.469446951953614189E-15, -1.000000000000000000 ) ) ;
#17530=ORIENTED_EDGE ( 'NONE', *, *, #11263, .F. ) ;
#17540=CARTESIAN_POINT ( 'NONE',  ( 0.000000000000000000, 0.000000000000000000, -50.00000000000000000 ) ) ;
#17554=CARTESIAN_POINT ( 'NONE',  ( -44.99999999999997868, -52.79999999999937899, 142.6500000000001478 ) ) ;
#17639=DIRECTION ( 'NONE',  ( -1.000000000000000000, -3.736327486719275871E-16, -0.000000000000000000 ) ) ;
#17670=ORIENTED_EDGE ( 'NONE', *, *, #8189, .F. ) ;
#17671=CARTESIAN_POINT ( 'NONE',  ( -65.00000000000000000, -52.79999999999933635, 155.0000000000001421 ) ) ;
#17739=ORIENTED_EDGE ( 'NONE', *, *, #23482, .T. ) ;
#17740=CARTESIAN_POINT ( 'NONE',  ( 25.00000000000002132, -52.79999999999930793, 155.0000000000001990 ) ) ;
#17743=ORIENTED_EDGE ( 'NONE', *, *, #1664, .F. ) ;
#17744=ADVANCED_FACE ( 'NONE', ( #10321, #16106, #13852 ), #21299, .T. ) ;
#17777=ORIENTED_EDGE ( 'NONE', *, *, #23000, .T. ) ;
#17778=EDGE_CURVE ( 'NONE', #13794, #10166, #4873, .T. ) ;
#17796=CARTESIAN_POINT ( 'NONE',  ( 45.00000000000002132, -52.79999999999936477, 140.0000000000001990 ) ) ;
#17801=ORIENTED_EDGE ( 'NONE', *, *, #3934, .F. ) ;
#17814=DIRECTION ( 'NONE',  ( 0.000000000000000000, 0.000000000000000000, 1.000000000000000000 ) ) ;
#17856=EDGE_LOOP ( 'NONE', ( #23206, #332, #13976, #700 ) ) ;
#17870=PLANE ( 'NONE',  #16671 ) ;
#17916=VERTEX_POINT ( 'NONE', #19835 ) ;
#17917=DIRECTION ( 'NONE',  ( 1.776356839400250465E-15, 1.000000000000000000, -3.392348130799088816E-15 ) ) ;
#17937=ORIENTED_EDGE ( 'NONE', *, *, #4761, .F. ) ;
#17948=EDGE_LOOP ( 'NONE', ( #6298, #4193, #17777, #5013 ) ) ;
#17963=VECTOR ( 'NONE', #13205, 1000.000000000000000 ) ;
#17991=FACE_OUTER_BOUND ( 'NONE', #2528, .T. ) ;
#17992=ORIENTED_EDGE ( 'NONE', *, *, #7406, .T. ) ;
#17997=ADVANCED_FACE ( 'NONE', ( #12766 ), #18255, .F. ) ;
#18024=DIRECTION ( 'NONE',  ( 0.000000000000000000, 0.000000000000000000, 1.000000000000000000 ) ) ;
#18052=ORIENTED_EDGE ( 'NONE', *, *, #1664, .T. ) ;
#18099=VECTOR ( 'NONE', #22093, 1000.000000000000000 ) ;
#18104=CARTESIAN_POINT ( 'NONE',  ( -44.99999999999997868, -56.79999999999937899, 140.0000000000001421 ) ) ;
#18116=AXIS2_PLACEMENT_3D ( 'NONE', #14569, #9130, #9490 ) ;
#18122=CARTESIAN_POINT ( 'NONE',  ( -64.99999999999998579, -56.79999999999943583, 125.0000000000001705 ) ) ;
#18231=CARTESIAN_POINT ( 'NONE',  ( 24.99999999999998579, 45.00100000000075084, 154.9999999999998579 ) ) ;
#18249=CYLINDRICAL_SURFACE ( 'NONE', #695, 10.00000000000000000 ) ;
#18255=CYLINDRICAL_SURFACE ( 'NONE', #20338, 2.649999999999985700 ) ;
#18262=CARTESIAN_POINT ( 'NONE',  ( 45.00000000000004974, -56.79999999999967031, 50.00000000000019895 ) ) ;
#18397=CARTESIAN_POINT ( 'NONE',  ( 0.000000000000000000, 0.000000000000000000, 20.00000000000000000 ) ) ;
#18412=LINE ( 'NONE', #20582, #21572 ) ;
#18423=EDGE_LOOP ( 'NONE', ( #22975, #15292 ) ) ;
#18432=VECTOR ( 'NONE', #22430, 1000.000000000000000 ) ;
#18478=LINE ( 'NONE', #14874, #12388 ) ;
#18502=ORIENTED_EDGE ( 'NONE', *, *, #1346, .F. ) ;
#18506=CARTESIAN_POINT ( 'NONE',  ( -64.99999999999997158, -52.79999999999974847, 35.00000000000017764 ) ) ;
#18567=DIRECTION ( 'NONE',  ( 0.000000000000000000, -2.618450529776326854E-15, -1.000000000000000000 ) ) ;
#18574=ORIENTED_EDGE ( 'NONE', *, *, #1443, .F. ) ;
#18606=VERTEX_POINT ( 'NONE', #4788 ) ;
#18619=VERTEX_POINT ( 'NONE', #12092 ) ;
#18663=CARTESIAN_POINT ( 'NONE',  ( -64.99999999999997158, -56.79999999999975557, 35.00000000000019185 ) ) ;
#18686=LINE ( 'NONE', #3853, #1425 ) ;
#18688=CARTESIAN_POINT ( 'NONE',  ( 0.000000000000000000, 0.000000000000000000, 169.9999999999999716 ) ) ;
#18762=FACE_BOUND ( 'NONE', #5695, .T. ) ;
#18795=FACE_OUTER_BOUND ( 'NONE', #8269, .T. ) ;
#18799=ORIENTED_EDGE ( 'NONE', *, *, #17311, .F. ) ;
#18825=VECTOR ( 'NONE', #6552, 1000.000000000000000 ) ;
#18970=FACE_OUTER_BOUND ( 'NONE', #3309, .T. ) ;
#18998=VERTEX_POINT ( 'NONE', #17554 ) ;
#19016=VERTEX_POINT ( 'NONE', #4880 ) ;
#19050=DIRECTION ( 'NONE',  ( 0.000000000000000000, -1.000000000000000000, 3.700743415417187942E-15 ) ) ;
#19089=ORIENTED_EDGE ( 'NONE', *, *, #19425, .F. ) ;
#19094=CARTESIAN_POINT ( 'NONE',  ( 65.00000000000004263, -52.79999999999959925, 65.00000000000018474 ) ) ;
#19096=AXIS2_PLACEMENT_3D ( 'NONE', #8103, #2766, #4818 ) ;
#19130=FACE_BOUND ( 'NONE', #6028, .T. ) ;
#19174=LINE ( 'NONE', #2637, #14950 ) ;
#19177=FACE_OUTER_BOUND ( 'NONE', #19491, .T. ) ;
#19183=ORIENTED_EDGE ( 'NONE', *, *, #2658, .T. ) ;
#19227=EDGE_CURVE ( 'NONE', #19560, #13294, #22924, .T. ) ;
#19235=APPLICATION_CONTEXT ( 'automotive_design' ) ;
#19246=AXIS2_PLACEMENT_3D ( 'NONE', #15515, #6673, #14067 ) ;
#19259=ORIENTED_EDGE ( 'NONE', *, *, #19759, .F. ) ;
#19281=EDGE_LOOP ( 'NONE', ( #11787, #16510, #15800, #1234 ) ) ;
#19292=ORIENTED_EDGE ( 'NONE', *, *, #8357, .F. ) ;
#19293=EDGE_LOOP ( 'NONE', ( #7510, #10875, #8563, #18502 ) ) ;
#19308=DIRECTION ( 'NONE',  ( -3.736327486719275871E-16, 1.000000000000000000, 0.000000000000000000 ) ) ;
#19324=ADVANCED_FACE ( 'NONE', ( #11642, #8109 ), #5911, .F. ) ;
#19327=ORIENTED_EDGE ( 'NONE', *, *, #7406, .F. ) ;
#19337=ORIENTED_EDGE ( 'NONE', *, *, #15885, .T. ) ;
#19374=ORIENTED_EDGE ( 'NONE', *, *, #7934, .T. ) ;
#19425=EDGE_CURVE ( 'NONE', #4511, #8574, #21727, .T. ) ;
#19433=CIRCLE ( 'NONE', #14456, 2.649999999999999467 ) ;
#19491=EDGE_LOOP ( 'NONE', ( #1324, #9565 ) ) ;
#19542=LINE ( 'NONE', #15844, #22677 ) ;
#19560=VERTEX_POINT ( 'NONE', #20732 ) ;
#19631=EDGE_CURVE ( 'NONE', #3415, #840, #9658, .T. ) ;
#19663=DIRECTION ( 'NONE',  ( 3.736327486719275871E-16, -1.000000000000000000, 3.469446951953614189E-15 ) ) ;
#19677=EDGE_CURVE ( 'NONE', #5510, #15457, #14122, .T. ) ;
#19687=ORIENTED_EDGE ( 'NONE', *, *, #10945, .F. ) ;
#19690=FACE_OUTER_BOUND ( 'NONE', #7658, .T. ) ;
#19697=CARTESIAN_POINT ( 'NONE',  ( -24.99999999999998934, 45.00100000000041689, 64.99999999999984368 ) ) ;
#19711=CARTESIAN_POINT ( 'NONE',  ( 0.000000000000000000, 0.000000000000000000, 169.9999999999999716 ) ) ;
#19741=DIRECTION ( 'NONE',  ( 0.000000000000000000, 1.000000000000000000, 0.000000000000000000 ) ) ;
#19759=EDGE_CURVE ( 'NONE', #10258, #10166, #4683, .T. ) ;
#19768=EDGE_CURVE ( 'NONE', #21871, #7027, #16534, .T. ) ;
#19797=( NAMED_UNIT ( * ) SI_UNIT ( $, .STERADIAN. ) SOLID_ANGLE_UNIT ( ) );
#19808=EDGE_CURVE ( 'NONE', #4703, #22432, #1865, .T. ) ;
#19810=ORIENTED_EDGE ( 'NONE', *, *, #19768, .T. ) ;
#19835=CARTESIAN_POINT ( 'NONE',  ( 45.00000000000000711, 5.510910596163090344E-15, 20.00000000000000000 ) ) ;
#19845=VECTOR ( 'NONE', #6691, 1000.000000000000000 ) ;
#19847=EDGE_LOOP ( 'NONE', ( #22968, #10907, #13212, #13023, #11623, #22761 ) ) ;
#19915=ORIENTED_EDGE ( 'NONE', *, *, #17353, .T. ) ;
#19916=VECTOR ( 'NONE', #15053, 1000.000000000000000 ) ;
#19936=ORIENTED_EDGE ( 'NONE', *, *, #17201, .T. ) ;
#19969=VERTEX_POINT ( 'NONE', #13522 ) ;
#19993=DIRECTION ( 'NONE',  ( -0.000000000000000000, 1.000000000000000000, -3.469446951953613794E-15 ) ) ;
#19995=CARTESIAN_POINT ( 'NONE',  ( -24.99999999999998934, 45.00100000000031031, 34.99999999999983658 ) ) ;
#19996=VECTOR ( 'NONE', #2614, 1000.000000000000000 ) ;
#20015=DIRECTION ( 'NONE',  ( 3.202566417187928841E-16, -1.000000000000000000, 3.469446951953614583E-15 ) ) ;
#20020=CARTESIAN_POINT ( 'NONE',  ( -44.99999999999995026, -52.79999999999969873, 50.00000000000018474 ) ) ;
#20031=VECTOR ( 'NONE', #9358, 1000.000000000000000 ) ;
#20050=VECTOR ( 'NONE', #16678, 1000.000000000000000 ) ;
#20071=LINE ( 'NONE', #11042, #3840 ) ;
#20080=CARTESIAN_POINT ( 'NONE',  ( -45.00000000000000711, 0.000000000000000000, 169.9999999999999716 ) ) ;
#20149=CIRCLE ( 'NONE', #109, 10.00000000000000000 ) ;
#20156=ORIENTED_EDGE ( 'NONE', *, *, #6661, .F. ) ;
#20160=ORIENTED_EDGE ( 'NONE', *, *, #60, .F. ) ;
#20219=ORIENTED_EDGE ( 'NONE', *, *, #14712, .T. ) ;
#20229=ORIENTED_EDGE ( 'NONE', *, *, #22341, .T. ) ;
#20243=EDGE_LOOP ( 'NONE', ( #16981, #23403, #2074, #7310, #23174, #7947, #11361, #8100 ) ) ;
#20269=DIRECTION ( 'NONE',  ( 0.000000000000000000, -1.000000000000000000, 3.469446951953614189E-15 ) ) ;
#20282=ORIENTED_EDGE ( 'NONE', *, *, #12859, .F. ) ;
#20338=AXIS2_PLACEMENT_3D ( 'NONE', #1707, #13470, #9569 ) ;
#20339=DIRECTION ( 'NONE',  ( 1.000000000000000000, 0.000000000000000000, 0.000000000000000000 ) ) ;
#20374=EDGE_LOOP ( 'NONE', ( #11337, #20229, #12872, #19292, #13909, #15104, #7740, #3681 ) ) ;
#20381=AXIS2_PLACEMENT_3D ( 'NONE', #6199, #22841, #6307 ) ;
#20382=AXIS2_PLACEMENT_3D ( 'NONE', #19711, #4640, #8868 ) ;
#20409=CARTESIAN_POINT ( 'NONE',  ( 65.00000000000005684, -52.79999999999970584, 35.00000000000017764 ) ) ;
#20431=CARTESIAN_POINT ( 'NONE',  ( 24.99999999999998579, 45.00100000000075084, 154.9999999999998579 ) ) ;
#20441=AXIS2_PLACEMENT_3D ( 'NONE', #23150, #11978, #21100 ) ;
#20465=EDGE_CURVE ( 'NONE', #19969, #21767, #14641, .T. ) ;
#20491=LINE ( 'NONE', #5884, #19996 ) ;
#20506=CARTESIAN_POINT ( 'NONE',  ( 45.00000000000002132, -52.79999999999936477, 140.0000000000001990 ) ) ;
#20529=AXIS2_PLACEMENT_3D ( 'NONE', #15951, #15845, #21131 ) ;
#20557=VECTOR ( 'NONE', #16350, 1000.000000000000000 ) ;
#20582=CARTESIAN_POINT ( 'NONE',  ( -64.99999999999998579, -52.79999999999942872, 125.0000000000001421 ) ) ;
#20585=( LENGTH_UNIT ( ) NAMED_UNIT ( * ) SI_UNIT ( .MILLI., .METRE. ) );
#20595=CARTESIAN_POINT ( 'NONE',  ( 0.000000000000000000, 0.000000000000000000, 169.9999999999999716 ) ) ;
#20598=FACE_BOUND ( 'NONE', #22447, .T. ) ;
#20609=DIRECTION ( 'NONE',  ( -0.000000000000000000, 1.000000000000000000, -3.469446951953613794E-15 ) ) ;
#20704=FACE_OUTER_BOUND ( 'NONE', #14373, .T. ) ;
#20732=CARTESIAN_POINT ( 'NONE',  ( -64.99999999999995737, -52.79999999999965610, 65.00000000000017053 ) ) ;
#20796=DIRECTION ( 'NONE',  ( 1.000000000000000000, 3.736327486719275871E-16, -1.296299001029869881E-30 ) ) ;
#20798=CARTESIAN_POINT ( 'NONE',  ( -44.99999999999997868, -52.79999999999937899, 142.6500000000001478 ) ) ;
#20812=ORIENTED_EDGE ( 'NONE', *, *, #1346, .T. ) ;
#20874=DIRECTION ( 'NONE',  ( -0.000000000000000000, 1.000000000000000000, -3.469446951953613794E-15 ) ) ;
#20893=DIRECTION ( 'NONE',  ( 3.469446951953614682E-16, -1.000000000000000000, 3.483493295888648978E-15 ) ) ;
#20915=CARTESIAN_POINT ( 'NONE',  ( -44.99999999999997868, -52.79999999999938609, 140.0000000000001421 ) ) ;
#20916=DIRECTION ( 'NONE',  ( -0.000000000000000000, 1.000000000000000000, -3.469446951953613794E-15 ) ) ;
#20919=CARTESIAN_POINT ( 'NONE',  ( 10.00000000000000000, 0.000000000000000000, -50.00000000000000000 ) ) ;
#20923=EDGE_LOOP ( 'NONE', ( #22226, #3786, #14091, #8895 ) ) ;
#20942=ORIENTED_EDGE ( 'NONE', *, *, #1344, .T. ) ;
#20944=DIRECTION ( 'NONE',  ( 0.000000000000000000, 0.000000000000000000, 1.000000000000000000 ) ) ;
#20953=VECTOR ( 'NONE', #15026, 1000.000000000000000 ) ;
#21077=ORIENTED_EDGE ( 'NONE', *, *, #23030, .F. ) ;
#21083=FACE_OUTER_BOUND ( 'NONE', #23785, .T. ) ;
#21100=DIRECTION ( 'NONE',  ( 4.625929269271498733E-16, 0.000000000000000000, 1.000000000000000000 ) ) ;
#21104=ADVANCED_FACE ( 'NONE', ( #797 ), #15546, .T. ) ;
#21124=LINE ( 'NONE', #17497, #7927 ) ;
#21125=DIRECTION ( 'NONE',  ( 1.000000000000000000, 3.736327486719275871E-16, -1.296299001029869881E-30 ) ) ;
#21127=ORIENTED_EDGE ( 'NONE', *, *, #23030, .T. ) ;
#21131=DIRECTION ( 'NONE',  ( 1.000000000000000000, 0.000000000000000000, -0.000000000000000000 ) ) ;
#21158=CARTESIAN_POINT ( 'NONE',  ( 0.000000000000000000, 0.000000000000000000, 35.00000000000000000 ) ) ;
#21165=COLOUR_RGB ( '',0.8941176470588234615, 0.8941176470588234615, 0.8941176470588234615 ) ;
#21174=FACE_OUTER_BOUND ( 'NONE', #21184, .T. ) ;
#21176=EDGE_CURVE ( 'NONE', #4246, #8364, #21549, .T. ) ;
#21179=DIRECTION ( 'NONE',  ( 0.000000000000000000, -3.469446951953613794E-15, -1.000000000000000000 ) ) ;
#21184=EDGE_LOOP ( 'NONE', ( #10938, #7397, #7043, #2941 ) ) ;
#21250=LINE ( 'NONE', #12477, #12587 ) ;
#21267=ORIENTED_EDGE ( 'NONE', *, *, #21561, .F. ) ;
#21271=CARTESIAN_POINT ( 'NONE',  ( -65.00000000000000000, -52.79999999999933635, 155.0000000000001421 ) ) ;
#21299=PLANE ( 'NONE',  #2206 ) ;
#21344=EDGE_LOOP ( 'NONE', ( #18574, #11832, #21771, #5881 ) ) ;
#21351=CARTESIAN_POINT ( 'NONE',  ( 25.00000000000001066, 45.00100000000043821, 64.99999999999984368 ) ) ;
#21370=VERTEX_POINT ( 'NONE', #23706 ) ;
#21371=LINE ( 'NONE', #4713, #10302 ) ;
#21376=VERTEX_POINT ( 'NONE', #3768 ) ;
#21387=VERTEX_POINT ( 'NONE', #1968 ) ;
#21415=VECTOR ( 'NONE', #8452, 1000.000000000000000 ) ;
#21416=LINE ( 'NONE', #17671, #19845 ) ;
#21419=ORIENTED_EDGE ( 'NONE', *, *, #3574, .F. ) ;
#21456=PLANE ( 'NONE',  #14816 ) ;
#21549=LINE ( 'NONE', #8527, #721 ) ;
#21561=EDGE_CURVE ( 'NONE', #17916, #12643, #5764, .T. ) ;
#21572=VECTOR ( 'NONE', #11451, 1000.000000000000000 ) ;
#21617=ORIENTED_EDGE ( 'NONE', *, *, #14844, .F. ) ;
#21625=CARTESIAN_POINT ( 'NONE',  ( 0.000000000000000000, 0.000000000000000000, 0.000000000000000000 ) ) ;
#21640=CARTESIAN_POINT ( 'NONE',  ( -45.00000000000000711, 0.000000000000000000, 20.00000000000000000 ) ) ;
#21643=CARTESIAN_POINT ( 'NONE',  ( -1.500000000000000000, 12.00000000000000000, 0.000000000000000000 ) ) ;
#21659=FACE_BOUND ( 'NONE', #10669, .T. ) ;
#21668=CARTESIAN_POINT ( 'NONE',  ( -64.99999999999995737, -56.79999999999964899, 65.00000000000018474 ) ) ;
#21711=DIRECTION ( 'NONE',  ( 0.000000000000000000, -2.618450529776313049E-15, -1.000000000000000000 ) ) ;
#21727=LINE ( 'NONE', #23045, #15812 ) ;
#21739=VERTEX_POINT ( 'NONE', #20409 ) ;
#21762=AXIS2_PLACEMENT_3D ( 'NONE', #2145, #4078, #19050 ) ;
#21767=VERTEX_POINT ( 'NONE', #5684 ) ;
#21771=ORIENTED_EDGE ( 'NONE', *, *, #3963, .T. ) ;
#21773=CARTESIAN_POINT ( 'NONE',  ( -24.99999999999998579, -37.41657386773942306, 125.0000000000001705 ) ) ;
#21827=DIRECTION ( 'NONE',  ( 0.000000000000000000, -2.618450529776326854E-15, -1.000000000000000000 ) ) ;
#21828=LINE ( 'NONE', #14731, #12906 ) ;
#21865=EDGE_LOOP ( 'NONE', ( #1593, #7017 ) ) ;
#21871=VERTEX_POINT ( 'NONE', #1895 ) ;
#21876=VECTOR ( 'NONE', #6685, 1000.000000000000000 ) ;
#21909=VECTOR ( 'NONE', #23253, 1000.000000000000000 ) ;
#21914=CARTESIAN_POINT ( 'NONE',  ( 25.00000000000001066, 45.00100000000043821, 64.99999999999984368 ) ) ;
#21940=VECTOR ( 'NONE', #9227, 1000.000000000000000 ) ;
#21943=ORIENTED_EDGE ( 'NONE', *, *, #10226, .T. ) ;
#21962=VECTOR ( 'NONE', #16481, 1000.000000000000000 ) ;
#21969=EDGE_CURVE ( 'NONE', #8692, #9373, #14564, .T. ) ;
#21992=CIRCLE ( 'NONE', #3382, 45.00000000000000711 ) ;
#22047=DIRECTION ( 'NONE',  ( 1.000000000000000000, -9.769962616701377556E-15, 0.000000000000000000 ) ) ;
#22060=DIRECTION ( 'NONE',  ( 3.202566417187928841E-16, -1.000000000000000000, 3.469446951953614583E-15 ) ) ;
#22065=DIRECTION ( 'NONE',  ( -0.000000000000000000, 1.000000000000000000, -3.469446951953613794E-15 ) ) ;
#22080=ORIENTED_EDGE ( 'NONE', *, *, #19227, .F. ) ;
#22093=DIRECTION ( 'NONE',  ( 0.000000000000000000, 0.000000000000000000, 1.000000000000000000 ) ) ;
#22096=LINE ( 'NONE', #2168, #15585 ) ;
#22174=DIRECTION ( 'NONE',  ( 3.469446951953614682E-16, -1.000000000000000000, 3.483493295888648978E-15 ) ) ;
#22193=UNCERTAINTY_MEASURE_WITH_UNIT (LENGTH_MEASURE( 1.000000000000000082E-05 ), #4714, 'distance_accuracy_value', 'NONE');
#22195=AXIS2_PLACEMENT_3D ( 'NONE', #18262, #3529, #22236 ) ;
#22201=CARTESIAN_POINT ( 'NONE',  ( -44.99999999999997868, -52.79999999999939320, 137.3500000000001648 ) ) ;
#22226=ORIENTED_EDGE ( 'NONE', *, *, #585, .F. ) ;
#22236=DIRECTION ( 'NONE',  ( 0.000000000000000000, -2.618450529776313049E-15, -1.000000000000000000 ) ) ;
#22256=ADVANCED_BREP_SHAPE_REPRESENTATION ( '', ( #12608, #11210 ), #7665 ) ;
#22258=LINE ( 'NONE', #16726, #21962 ) ;
#22273=CARTESIAN_POINT ( 'NONE',  ( -24.99999999999995381, -52.79999999999975557, 35.00000000000017764 ) ) ;
#22290=VECTOR ( 'NONE', #7379, 1000.000000000000000 ) ;
#22316=VECTOR ( 'NONE', #7400, 1000.000000000000000 ) ;
#22317=CIRCLE ( 'NONE', #13874, 2.649999999999999467 ) ;
#22319=ORIENTED_EDGE ( 'NONE', *, *, #267, .F. ) ;
#22341=EDGE_CURVE ( 'NONE', #4703, #19969, #21992, .T. ) ;
#22356=VECTOR ( 'NONE', #13971, 1000.000000000000000 ) ;
#22364=LINE ( 'NONE', #11408, #15804 ) ;
#22430=DIRECTION ( 'NONE',  ( 1.000000000000000000, 3.736327486719276364E-16, 1.067522139062650425E-16 ) ) ;
#22432=VERTEX_POINT ( 'NONE', #12427 ) ;
#22447=EDGE_LOOP ( 'NONE', ( #9134, #3234 ) ) ;
#22450=ORIENTED_EDGE ( 'NONE', *, *, #6978, .F. ) ;
#22462=AXIS2_PLACEMENT_3D ( 'NONE', #7953, #20874, #6139 ) ;
#22482=ORIENTED_EDGE ( 'NONE', *, *, #4746, .F. ) ;
#22514=PLANE ( 'NONE',  #5937 ) ;
#22598=VERTEX_POINT ( 'NONE', #10838 ) ;
#22599=LINE ( 'NONE', #20798, #3594 ) ;
#22663=ORIENTED_EDGE ( 'NONE', *, *, #19631, .T. ) ;
#22664=CARTESIAN_POINT ( 'NONE',  ( 65.00000000000004263, -56.79999999999959925, 65.00000000000019895 ) ) ;
#22672=CARTESIAN_POINT ( 'NONE',  ( -44.99999999999997868, -56.79999999999938609, 137.3500000000001648 ) ) ;
#22677=VECTOR ( 'NONE', #418, 1000.000000000000000 ) ;
#22679=FACE_OUTER_BOUND ( 'NONE', #22746, .T. ) ;
#22707=EDGE_CURVE ( 'NONE', #17333, #5510, #19542, .T. ) ;
#22727=CARTESIAN_POINT ( 'NONE',  ( 45.00000000000002132, -52.79999999999935767, 142.6500000000002046 ) ) ;
#22728=ORIENTED_EDGE ( 'NONE', *, *, #11663, .F. ) ;
#22746=EDGE_LOOP ( 'NONE', ( #15678, #6499, #6524, #12006 ) ) ;
#22761=ORIENTED_EDGE ( 'NONE', *, *, #23452, .F. ) ;
#22783=CARTESIAN_POINT ( 'NONE',  ( -1.500000000000000000, 0.000000000000000000, 0.000000000000000000 ) ) ;
#22841=DIRECTION ( 'NONE',  ( -0.000000000000000000, 1.000000000000000000, -3.469446951953613794E-15 ) ) ;
#22887=CIRCLE ( 'NONE', #2057, 2.649999999999985700 ) ;
#22889=DIRECTION ( 'NONE',  ( 0.000000000000000000, -1.000000000000000000, -0.000000000000000000 ) ) ;
#22911=VECTOR ( 'NONE', #10904, 1000.000000000000000 ) ;
#22924=LINE ( 'NONE', #6396, #10830 ) ;
#22968=ORIENTED_EDGE ( 'NONE', *, *, #7230, .F. ) ;
#22975=ORIENTED_EDGE ( 'NONE', *, *, #16136, .F. ) ;
#22989=EDGE_CURVE ( 'NONE', #22432, #12588, #347, .T. ) ;
#23000=EDGE_CURVE ( 'NONE', #21376, #21387, #11152, .T. ) ;
#23013=CARTESIAN_POINT ( 'NONE',  ( 45.00000000000004974, -52.79999999999967031, 50.00000000000018474 ) ) ;
#23030=EDGE_CURVE ( 'NONE', #2982, #13294, #9173, .T. ) ;
#23045=CARTESIAN_POINT ( 'NONE',  ( -44.99999999999995026, -52.79999999999970584, 47.35000000000018616 ) ) ;
#23065=VECTOR ( 'NONE', #12096, 1000.000000000000000 ) ;
#23088=LINE ( 'NONE', #6564, #22356 ) ;
#23094=FACE_OUTER_BOUND ( 'NONE', #14264, .T. ) ;
#23150=CARTESIAN_POINT ( 'NONE',  ( 65.00000000000001421, -52.79999999999938609, 125.0000000000002274 ) ) ;
#23163=ORIENTED_EDGE ( 'NONE', *, *, #13645, .F. ) ;
#23174=ORIENTED_EDGE ( 'NONE', *, *, #60, .T. ) ;
#23197=FACE_OUTER_BOUND ( 'NONE', #2437, .T. ) ;
#23206=ORIENTED_EDGE ( 'NONE', *, *, #5579, .F. ) ;
#23222=AXIS2_PLACEMENT_3D ( 'NONE', #16329, #23790, #2045 ) ;
#23240=VECTOR ( 'NONE', #12842, 1000.000000000000000 ) ;
#23246=CARTESIAN_POINT ( 'NONE',  ( 65.00000000000004263, -56.79999999999959925, 65.00000000000019895 ) ) ;
#23252=ORIENTED_EDGE ( 'NONE', *, *, #22989, .T. ) ;
#23253=DIRECTION ( 'NONE',  ( -4.625929269271485914E-16, -3.469446951953614583E-15, -1.000000000000000000 ) ) ;
#23296=CARTESIAN_POINT ( 'NONE',  ( 25.00000000000001421, -37.41657386773940885, 155.0000000000001990 ) ) ;
#23305=EDGE_LOOP ( 'NONE', ( #8596, #6271, #2679, #17743 ) ) ;
#23309=VERTEX_POINT ( 'NONE', #1180 ) ;
#23320=VECTOR ( 'NONE', #7101, 1000.000000000000000 ) ;
#23327=VECTOR ( 'NONE', #16543, 1000.000000000000000 ) ;
#23331=FACE_OUTER_BOUND ( 'NONE', #17948, .T. ) ;
#23333=ADVANCED_FACE ( 'NONE', ( #12683 ), #16155, .F. ) ;
#23358=LINE ( 'NONE', #4531, #14801 ) ;
#23403=ORIENTED_EDGE ( 'NONE', *, *, #13629, .T. ) ;
#23428=CARTESIAN_POINT ( 'NONE',  ( 10.00000000000000000, 0.000000000000000000, 20.00000000000000000 ) ) ;
#23433=( LENGTH_UNIT ( ) NAMED_UNIT ( * ) SI_UNIT ( .MILLI., .METRE. ) );
#23452=EDGE_CURVE ( 'NONE', #8832, #13544, #12349, .T. ) ;
#23458=AXIS2_PLACEMENT_3D ( 'NONE', #8647, #3189, #2836 ) ;
#23474=CIRCLE ( 'NONE', #6959, 10.00000000000000000 ) ;
#23482=EDGE_CURVE ( 'NONE', #15472, #11870, #13038, .T. ) ;
#23493=EDGE_CURVE ( 'NONE', #23309, #14920, #18412, .T. ) ;
#23523=DIRECTION ( 'NONE',  ( -1.000000000000000000, -3.202566417187951028E-16, -6.405132834375902056E-16 ) ) ;
#23551=DIRECTION ( 'NONE',  ( 3.469446951953614682E-16, -1.000000000000000000, 3.483493295888648978E-15 ) ) ;
#23584=VERTEX_POINT ( 'NONE', #10114 ) ;
#23590=ORIENTED_EDGE ( 'NONE', *, *, #7394, .F. ) ;
#23605=AXIS2_PLACEMENT_3D ( 'NONE', #7571, #22060, #12938 ) ;
#23642=CARTESIAN_POINT ( 'NONE',  ( -44.99999999999995026, -52.79999999999969162, 52.65000000000018332 ) ) ;
#23697=DIRECTION ( 'NONE',  ( 3.469446951953614682E-16, -1.000000000000000000, 3.483493295888648978E-15 ) ) ;
#23706=CARTESIAN_POINT ( 'NONE',  ( -44.99999999999995026, -56.79999999999969162, 52.65000000000019753 ) ) ;
#23717=CARTESIAN_POINT ( 'NONE',  ( 65.00000000000005684, -56.79999999999970584, 35.00000000000019185 ) ) ;
#23718=VECTOR ( 'NONE', #2465, 1000.000000000000000 ) ;
#23738=ORIENTED_EDGE ( 'NONE', *, *, #3538, .F. ) ;
#23754=CARTESIAN_POINT ( 'NONE',  ( -65.00000000000000000, -52.79999999999933635, 155.0000000000001421 ) ) ;
#23779=CIRCLE ( 'NONE', #13044, 2.649999999999992806 ) ;
#23785=EDGE_LOOP ( 'NONE', ( #5195, #20942, #4804, #17801 ) ) ;
#23790=DIRECTION ( 'NONE',  ( -0.000000000000000000, 1.000000000000000000, -3.469446951953613794E-15 ) ) ;
#23928=COLOUR_RGB('Off White',0.89,0.88,0.83);
#23929=FILL_AREA_STYLE_COLOUR('',#23928);
#23930=FILL_AREA_STYLE('',(#23929));
#23931=SURFACE_STYLE_FILL_AREA(#23930);
#23932=SURFACE_SIDE_STYLE('',(#23931));
#23933=SURFACE_STYLE_USAGE(.BOTH.,#23932);
#23934=PRESENTATION_STYLE_ASSIGNMENT((#23933));
ENDSEC;
END-ISO-10303-21;
